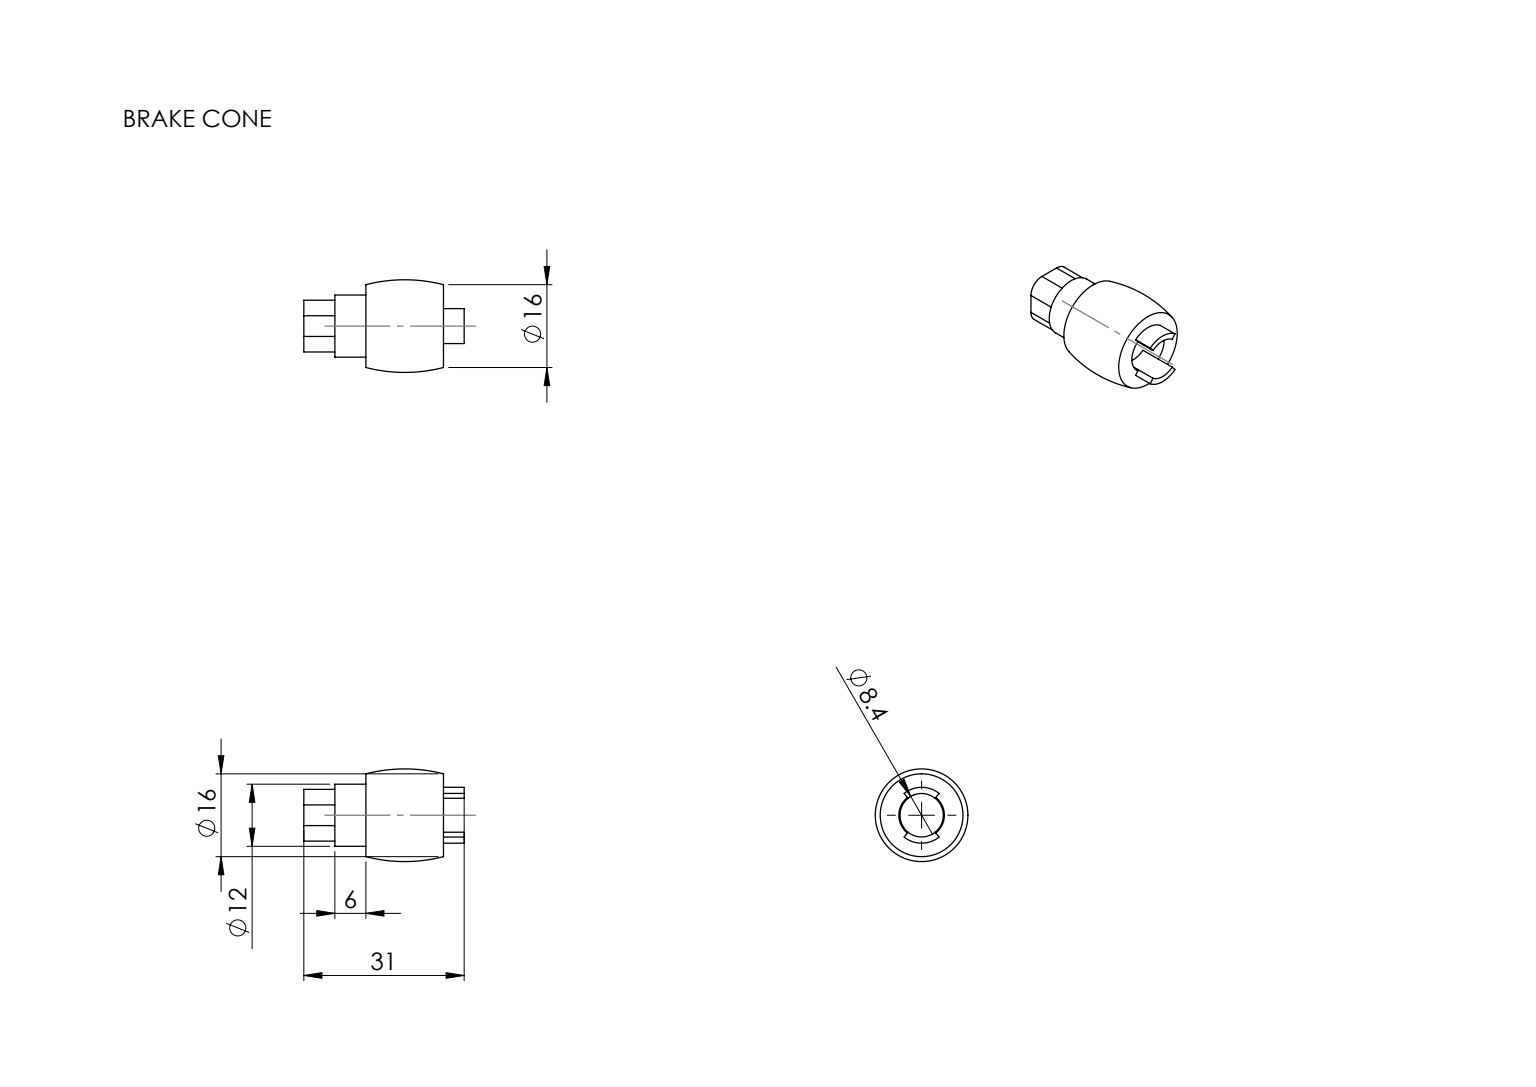
ISO-10303-21;
HEADER;
FILE_DESCRIPTION (('STEP AP214'),
    '1' );
FILE_NAME ('brake cone.step',
    '2026-10-08T05:56:58',
    ( '' ),
    ( '' ),
    'SwSTEP 2.0',
    'SolidWorks 2026',
    '' );
FILE_SCHEMA (( 'AUTOMOTIVE_DESIGN' ));
ENDSEC;

DATA;
#3=AXIS2_PLACEMENT_3D ( 'NONE', #18095, #1186, #4385 ) ;
#13=CARTESIAN_POINT ( 'NONE',  ( -15.00000000000000355, 4.874999999999997335, -3.903123748999000053 ) ) ;
#14=ADVANCED_FACE ( 'NONE', ( #14340, #12840 ), #18938, .T. ) ;
#25=CYLINDRICAL_SURFACE ( 'NONE', #12194, 5.400000000000000355 ) ;
#29=CARTESIAN_POINT ( 'NONE',  ( -41.99999999999999289, -2.000000000000001776, 5.000000000000000000 ) ) ;
#46=VECTOR ( 'NONE', #13444, 1000.000000000000000 ) ;
#90=PLANE ( 'NONE',  #2084 ) ;
#96=ORIENTED_EDGE ( 'NONE', *, *, #17923, .T. ) ;
#107=EDGE_LOOP ( 'NONE', ( #13060, #5147, #11835, #11833, #16317, #5831 ) ) ;
#112=EDGE_LOOP ( 'NONE', ( #14976, #17083 ) ) ;
#123=VERTEX_POINT ( 'NONE', #15646 ) ;
#140=LINE ( 'NONE', #6221, #2071 ) ;
#166=ORIENTED_EDGE ( 'NONE', *, *, #11587, .F. ) ;
#170=EDGE_CURVE ( 'NONE', #2370, #11052, #11954, .T. ) ;
#178=LINE ( 'NONE', #6262, #6325 ) ;
#190=EDGE_CURVE ( 'NONE', #10991, #3279, #7426, .T. ) ;
#207=CARTESIAN_POINT ( 'NONE',  ( -41.99999999999999289, -2.000000000000001776, -2.000000000000000000 ) ) ;
#240=DIRECTION ( 'NONE',  ( 0.000000000000000000, 0.000000000000000000, 1.000000000000000000 ) ) ;
#251=AXIS2_PLACEMENT_3D ( 'NONE', #17536, #9945, #11526 ) ;
#315=ORIENTED_EDGE ( 'NONE', *, *, #13010, .T. ) ;
#337=DIRECTION ( 'NONE',  ( 1.000000000000000000, 6.419766481290786633E-33, -0.000000000000000000 ) ) ;
#348=ORIENTED_EDGE ( 'NONE', *, *, #8508, .T. ) ;
#359=CARTESIAN_POINT ( 'NONE',  ( -11.00000000000000355, -4.215373648918917304, -3.375000000000002665 ) ) ;
#371=ADVANCED_FACE ( 'NONE', ( #7931 ), #17448, .F. ) ;
#385=EDGE_CURVE ( 'NONE', #2370, #813, #18633, .T. ) ;
#410=CIRCLE ( 'NONE', #17678, 5.400000000000000355 ) ;
#413=ADVANCED_FACE ( 'NONE', ( #6417 ), #18643, .T. ) ;
#438=PLANE ( 'NONE',  #10003 ) ;
#452=DIRECTION ( 'NONE',  ( 0.000000000000000000, 1.000000000000000000, 0.000000000000000000 ) ) ;
#464=ORIENTED_EDGE ( 'NONE', *, *, #491, .T. ) ;
#467=AXIS2_PLACEMENT_3D ( 'NONE', #2237, #17453, #19046 ) ;
#470=PLANE ( 'NONE',  #17230 ) ;
#483=DIRECTION ( 'NONE',  ( -1.000000000000000000, -6.419766481290786633E-33, 0.000000000000000000 ) ) ;
#491=EDGE_CURVE ( 'NONE', #14026, #12070, #7010, .T. ) ;
#504=EDGE_CURVE ( 'NONE', #17943, #9399, #4719, .T. ) ;
#516=ORIENTED_EDGE ( 'NONE', *, *, #190, .T. ) ;
#527=EDGE_CURVE ( 'NONE', #16516, #11599, #15232, .T. ) ;
#530=VERTEX_POINT ( 'NONE', #15333 ) ;
#559=FACE_BOUND ( 'NONE', #1659, .T. ) ;
#561=EDGE_LOOP ( 'NONE', ( #1766, #13669, #6712, #18454, #1075, #7563, #16391, #5040 ) ) ;
#565=VECTOR ( 'NONE', #8267, 1000.000000000000000 ) ;
#573=DIRECTION ( 'NONE',  ( 1.000000000000000000, 6.419766481290786633E-33, -0.000000000000000000 ) ) ;
#579=ORIENTED_EDGE ( 'NONE', *, *, #19561, .F. ) ;
#610=ORIENTED_EDGE ( 'NONE', *, *, #19296, .F. ) ;
#617=DIRECTION ( 'NONE',  ( 1.000000000000000000, 6.419766481290786633E-33, -0.000000000000000000 ) ) ;
#640=ADVANCED_FACE ( 'NONE', ( #14022 ), #1910, .T. ) ;
#644=ORIENTED_EDGE ( 'NONE', *, *, #6204, .T. ) ;
#655=ORIENTED_EDGE ( 'NONE', *, *, #19266, .F. ) ;
#702=DIRECTION ( 'NONE',  ( 6.419766481290786633E-33, -1.000000000000000000, 0.000000000000000000 ) ) ;
#708=ORIENTED_EDGE ( 'NONE', *, *, #12930, .T. ) ;
#727=ORIENTED_EDGE ( 'NONE', *, *, #2944, .F. ) ;
#766=SURFACE_STYLE_FILL_AREA ( #5055 ) ;
#767=PRODUCT_DEFINITION_SHAPE ( 'NONE', 'NONE',  #9076 ) ;
#776=EDGE_LOOP ( 'NONE', ( #15679, #8898, #8555, #10719 ) ) ;
#777=EDGE_CURVE ( 'NONE', #2407, #17288, #6813, .T. ) ;
#784=LINE ( 'NONE', #5274, #11574 ) ;
#813=VERTEX_POINT ( 'NONE', #13020 ) ;
#818=DIRECTION ( 'NONE',  ( 1.000000000000000000, 6.419766481290786633E-33, -0.000000000000000000 ) ) ;
#830=FACE_OUTER_BOUND ( 'NONE', #14532, .T. ) ;
#843=ORIENTED_EDGE ( 'NONE', *, *, #491, .F. ) ;
#885=DIRECTION ( 'NONE',  ( 1.000000000000000000, 1.224646799147353207E-16, 0.000000000000000000 ) ) ;
#913=DIRECTION ( 'NONE',  ( -1.000000000000000000, 1.224646799147353207E-16, 0.000000000000000000 ) ) ;
#920=FACE_OUTER_BOUND ( 'NONE', #18601, .T. ) ;
#927=CARTESIAN_POINT ( 'NONE',  ( -11.00000000000000355, 3.278623949159159778, 2.625000000000000888 ) ) ;
#951=ORIENTED_EDGE ( 'NONE', *, *, #13359, .T. ) ;
#952=CARTESIAN_POINT ( 'NONE',  ( -36.00000000000000000, 1.999999999999998224, -5.000000000000000000 ) ) ;
#957=EDGE_LOOP ( 'NONE', ( #10118, #13966, #3448, #4840 ) ) ;
#973=CIRCLE ( 'NONE', #3, 3.000000000000000000 ) ;
#1030=ORIENTED_EDGE ( 'NONE', *, *, #6750, .F. ) ;
#1040=CARTESIAN_POINT ( 'NONE',  ( -10.99900000000000233, 4.200000000000000178, 5.143516556418882928E-16 ) ) ;
#1044=FACE_OUTER_BOUND ( 'NONE', #18531, .T. ) ;
#1075=ORIENTED_EDGE ( 'NONE', *, *, #15150, .T. ) ;
#1083=DIRECTION ( 'NONE',  ( -1.000000000000000000, -1.224646799147353207E-16, 0.000000000000000000 ) ) ;
#1109=CARTESIAN_POINT ( 'NONE',  ( -19.00000000000000355, -4.200000000000000178, 0.000000000000000000 ) ) ;
#1111=ORIENTED_EDGE ( 'NONE', *, *, #11893, .T. ) ;
#1186=DIRECTION ( 'NONE',  ( -1.000000000000000000, 0.000000000000000000, 0.000000000000000000 ) ) ;
#1242=( NAMED_UNIT ( * ) PLANE_ANGLE_UNIT ( ) SI_UNIT ( $, .RADIAN. ) );
#1243=PRODUCT ( 'brake cone', 'brake cone', '', ( #7842 ) ) ;
#1244=VECTOR ( 'NONE', #3600, 1000.000000000000000 ) ;
#1246=LINE ( 'NONE', #7323, #46 ) ;
#1283=ORIENTED_EDGE ( 'NONE', *, *, #10304, .T. ) ;
#1295=EDGE_CURVE ( 'NONE', #5646, #11950, #19297, .T. ) ;
#1330=ORIENTED_EDGE ( 'NONE', *, *, #12486, .F. ) ;
#1362=ORIENTED_EDGE ( 'NONE', *, *, #16739, .T. ) ;
#1371=DIRECTION ( 'NONE',  ( 9.559896011775280412E-17, -0.7806247497997995666, -0.6250000000000001110 ) ) ;
#1395=DIRECTION ( 'NONE',  ( -1.000000000000000000, -6.419766481290788001E-33, -0.000000000000000000 ) ) ;
#1414=EDGE_CURVE ( 'NONE', #16293, #11503, #18340, .T. ) ;
#1469=VECTOR ( 'NONE', #9851, 1000.000000000000114 ) ;
#1491=CARTESIAN_POINT ( 'NONE',  ( -41.99999999999999289, -5.000000000000001776, 5.000000000000000000 ) ) ;
#1493=ORIENTED_EDGE ( 'NONE', *, *, #19398, .T. ) ;
#1508=VECTOR ( 'NONE', #13779, 1000.000000000000000 ) ;
#1516=CARTESIAN_POINT ( 'NONE',  ( -15.00000000000000355, 4.215373648918918192, 3.375000000000000888 ) ) ;
#1534=DIRECTION ( 'NONE',  ( -1.000000000000000000, 1.224646799147353207E-16, 0.000000000000000000 ) ) ;
#1539=CIRCLE ( 'NONE', #12081, 4.200000000000000178 ) ;
#1572=ORIENTED_EDGE ( 'NONE', *, *, #4535, .T. ) ;
#1581=CARTESIAN_POINT ( 'NONE',  ( -36.00000000000000000, 1.999999999999999112, -2.000000000000000000 ) ) ;
#1588=FACE_OUTER_BOUND ( 'NONE', #2951, .T. ) ;
#1623=DIRECTION ( 'NONE',  ( 7.654042494670959086E-17, 0.6250000000000002220, 0.7806247497997996776 ) ) ;
#1659=EDGE_LOOP ( 'NONE', ( #3254, #3461 ) ) ;
#1676=SHAPE_REPRESENTATION_RELATIONSHIP ( 'NONE' , 'NONE' ,  #12077, #3271 ) ;
#1679=LINE ( 'NONE', #3474, #4102 ) ;
#1685=DIRECTION ( 'NONE',  ( -1.000000000000000000, -6.419766481290786633E-33, 0.000000000000000000 ) ) ;
#1693=ADVANCED_FACE ( 'NONE', ( #11331 ), #17129, .F. ) ;
#1716=DIRECTION ( 'NONE',  ( -1.000000000000000000, 1.224646799147353207E-16, 0.000000000000000000 ) ) ;
#1745=ORIENTED_EDGE ( 'NONE', *, *, #18107, .T. ) ;
#1754=LINE ( 'NONE', #13958, #6782 ) ;
#1766=ORIENTED_EDGE ( 'NONE', *, *, #12191, .T. ) ;
#1860=CIRCLE ( 'NONE', #15588, 5.400000000000000355 ) ;
#1867=ORIENTED_EDGE ( 'NONE', *, *, #12851, .F. ) ;
#1870=ORIENTED_EDGE ( 'NONE', *, *, #7757, .T. ) ;
#1882=ORIENTED_EDGE ( 'NONE', *, *, #16897, .T. ) ;
#1887=EDGE_CURVE ( 'NONE', #11052, #6746, #3980, .T. ) ;
#1892=DIRECTION ( 'NONE',  ( -1.000000000000000000, -6.419766481290788001E-33, -0.000000000000000000 ) ) ;
#1902=ORIENTED_EDGE ( 'NONE', *, *, #2961, .T. ) ;
#1907=EDGE_LOOP ( 'NONE', ( #6125, #4723, #348, #7790 ) ) ;
#1910=PLANE ( 'NONE',  #12696 ) ;
#1917=CARTESIAN_POINT ( 'NONE',  ( -11.00000000000000355, 3.278623949159158446, -2.625000000000002220 ) ) ;
#1921=AXIS2_PLACEMENT_3D ( 'NONE', #14124, #1623, #3423 ) ;
#2002=EDGE_CURVE ( 'NONE', #17554, #17936, #16514, .T. ) ;
#2009=VERTEX_POINT ( 'NONE', #8907 ) ;
#2010=AXIS2_PLACEMENT_3D ( 'NONE', #9492, #11283, #11182 ) ;
#2015=LINE ( 'NONE', #14223, #10652 ) ;
#2020=ORIENTED_EDGE ( 'NONE', *, *, #13795, .F. ) ;
#2045=DIRECTION ( 'NONE',  ( -1.000000000000000000, 1.224646799147353207E-16, 0.000000000000000000 ) ) ;
#2061=ORIENTED_EDGE ( 'NONE', *, *, #19767, .F. ) ;
#2065=ORIENTED_EDGE ( 'NONE', *, *, #7779, .F. ) ;
#2071=VECTOR ( 'NONE', #13745, 1000.000000000000000 ) ;
#2076=CARTESIAN_POINT ( 'NONE',  ( -19.00000000000000355, 4.400000000000000355, 0.000000000000000000 ) ) ;
#2084=AXIS2_PLACEMENT_3D ( 'NONE', #7784, #6179, #12691 ) ;
#2122=VECTOR ( 'NONE', #4317, 1000.000000000000000 ) ;
#2130=ADVANCED_FACE ( 'NONE', ( #11197 ), #9711, .F. ) ;
#2152=CIRCLE ( 'NONE', #17170, 5.400000000000000355 ) ;
#2171=CARTESIAN_POINT ( 'NONE',  ( -41.99999999999999289, -1.469576158976823947E-15, 0.000000000000000000 ) ) ;
#2232=ORIENTED_EDGE ( 'NONE', *, *, #11453, .T. ) ;
#2237=CARTESIAN_POINT ( 'NONE',  ( -11.00000000000000355, 4.898587196589412829E-16, 0.000000000000000000 ) ) ;
#2247=ORIENTED_EDGE ( 'NONE', *, *, #19398, .F. ) ;
#2278=AXIS2_PLACEMENT_3D ( 'NONE', #13838, #18436, #19734 ) ;
#2282=DIRECTION ( 'NONE',  ( 1.000000000000000000, 6.419766481290786633E-33, -0.000000000000000000 ) ) ;
#2291=AXIS2_PLACEMENT_3D ( 'NONE', #6294, #6200, #11114 ) ;
#2347=DIRECTION ( 'NONE',  ( 0.000000000000000000, -1.000000000000000000, 0.000000000000000000 ) ) ;
#2365=VERTEX_POINT ( 'NONE', #9087 ) ;
#2370=VERTEX_POINT ( 'NONE', #12181 ) ;
#2407=VERTEX_POINT ( 'NONE', #8786 ) ;
#2413=AXIS2_PLACEMENT_3D ( 'NONE', #11245, #7837, #4842 ) ;
#2460=DIRECTION ( 'NONE',  ( -1.000000000000000000, 0.000000000000000000, 0.000000000000000000 ) ) ;
#2468=DIRECTION ( 'NONE',  ( 0.000000000000000000, 1.000000000000000000, 0.000000000000000000 ) ) ;
#2479=CIRCLE ( 'NONE', #251, 30.00000000000000355 ) ;
#2491=AXIS2_PLACEMENT_3D ( 'NONE', #6337, #3251, #18656 ) ;
#2508=AXIS2_PLACEMENT_3D ( 'NONE', #4240, #10254, #2629 ) ;
#2511=PLANE ( 'NONE',  #16664 ) ;
#2516=FACE_OUTER_BOUND ( 'NONE', #16831, .T. ) ;
#2525=DIRECTION ( 'NONE',  ( 1.000000000000000000, 6.419766481290786633E-33, -0.000000000000000000 ) ) ;
#2539=ORIENTED_EDGE ( 'NONE', *, *, #7560, .T. ) ;
#2548=ORIENTED_EDGE ( 'NONE', *, *, #15430, .F. ) ;
#2628=DIRECTION ( 'NONE',  ( -1.000000000000000000, -6.419766481290788001E-33, -0.000000000000000000 ) ) ;
#2629=DIRECTION ( 'NONE',  ( 0.000000000000000000, -1.000000000000000000, 0.000000000000000000 ) ) ;
#2739=CARTESIAN_POINT ( 'NONE',  ( -30.00000000000000000, 8.000000000000000000, 0.000000000000000000 ) ) ;
#2792=DIRECTION ( 'NONE',  ( -9.559896011775280412E-17, -0.7806247497997995666, -0.6250000000000002220 ) ) ;
#2839=DIRECTION ( 'NONE',  ( -1.000000000000000000, -1.224646799147353207E-16, -0.000000000000000000 ) ) ;
#2871=ORIENTED_EDGE ( 'NONE', *, *, #19538, .F. ) ;
#2889=EDGE_CURVE ( 'NONE', #123, #9264, #1754, .T. ) ;
#2891=PLANE ( 'NONE',  #3067 ) ;
#2905=AXIS2_PLACEMENT_3D ( 'NONE', #15793, #8184, #13348 ) ;
#2933=ADVANCED_FACE ( 'NONE', ( #559, #3747 ), #6928, .T. ) ;
#2944=EDGE_CURVE ( 'NONE', #12101, #5745, #3928, .T. ) ;
#2951=EDGE_LOOP ( 'NONE', ( #1493, #13570, #18839, #2548, #13326, #16612 ) ) ;
#2961=EDGE_CURVE ( 'NONE', #17554, #3802, #14354, .T. ) ;
#2972=DIRECTION ( 'NONE',  ( -1.000000000000000000, -6.419766481290786633E-33, 0.000000000000000000 ) ) ;
#3019=VERTEX_POINT ( 'NONE', #6092 ) ;
#3067=AXIS2_PLACEMENT_3D ( 'NONE', #10511, #19606, #13503 ) ;
#3085=CIRCLE ( 'NONE', #14277, 3.000000000000000000 ) ;
#3105=CARTESIAN_POINT ( 'NONE',  ( -41.99999999999999289, 1.999999999999998224, -2.000000000000000000 ) ) ;
#3137=CARTESIAN_POINT ( 'NONE',  ( -19.00000000000000355, 3.278623949159158890, 2.625000000000000888 ) ) ;
#3142=CIRCLE ( 'NONE', #16246, 3.000000000000000000 ) ;
#3170=( NAMED_UNIT ( * ) PLANE_ANGLE_UNIT ( ) SI_UNIT ( $, .RADIAN. ) );
#3173=EDGE_LOOP ( 'NONE', ( #1745, #9621 ) ) ;
#3204=TOROIDAL_SURFACE ( 'NONE', #13424, -21.04737509655562988, 30.00000000000000355 ) ;
#3222=VERTEX_POINT ( 'NONE', #10297 ) ;
#3251=DIRECTION ( 'NONE',  ( -1.000000000000000000, 1.224646799147353207E-16, 0.000000000000000000 ) ) ;
#3254=ORIENTED_EDGE ( 'NONE', *, *, #10304, .F. ) ;
#3257=EDGE_LOOP ( 'NONE', ( #4050, #7202 ) ) ;
#3271=ADVANCED_BREP_SHAPE_REPRESENTATION ( '', ( #9200, #16724 ), #3651 ) ;
#3279=VERTEX_POINT ( 'NONE', #10008 ) ;
#3294=AXIS2_PLACEMENT_3D ( 'NONE', #3737, #8138, #15948 ) ;
#3301=CARTESIAN_POINT ( 'NONE',  ( -36.00000000000000000, -2.000000000000000888, -2.000000000000000000 ) ) ;
#3312=ORIENTED_EDGE ( 'NONE', *, *, #8331, .T. ) ;
#3322=DIRECTION ( 'NONE',  ( 1.000000000000000000, 6.419766481290786633E-33, -0.000000000000000000 ) ) ;
#3327=ORIENTED_EDGE ( 'NONE', *, *, #5451, .F. ) ;
#3379=CIRCLE ( 'NONE', #14252, 4.400000000000000355 ) ;
#3416=CARTESIAN_POINT ( 'NONE',  ( -19.00000000000000355, -4.898587196589412829E-16, 0.000000000000000000 ) ) ;
#3423=DIRECTION ( 'NONE',  ( 0.000000000000000000, -0.7806247497997995666, 0.6250000000000001110 ) ) ;
#3438=VECTOR ( 'NONE', #5443, 1000.000000000000000 ) ;
#3439=DIRECTION ( 'NONE',  ( 6.419766481290786633E-33, -1.000000000000000000, 0.000000000000000000 ) ) ;
#3440=DIRECTION ( 'NONE',  ( 0.000000000000000000, 1.000000000000000000, 0.000000000000000000 ) ) ;
#3442=ORIENTED_EDGE ( 'NONE', *, *, #8852, .T. ) ;
#3448=ORIENTED_EDGE ( 'NONE', *, *, #18107, .F. ) ;
#3458=EDGE_CURVE ( 'NONE', #3222, #14330, #2152, .T. ) ;
#3461=ORIENTED_EDGE ( 'NONE', *, *, #13010, .F. ) ;
#3469=SURFACE_STYLE_USAGE ( .BOTH. , #14173 ) ;
#3474=CARTESIAN_POINT ( 'NONE',  ( -41.99999999999999289, -5.000000000000001776, -2.000000000000000000 ) ) ;
#3478=PRODUCT_DEFINITION_FORMATION_WITH_SPECIFIED_SOURCE ( 'ANY', '', #1243, .NOT_KNOWN. ) ;
#3492=EDGE_LOOP ( 'NONE', ( #1111, #2539, #14378, #7011, #7147, #2065 ) ) ;
#3509=EDGE_LOOP ( 'NONE', ( #2020, #10777, #464, #19765 ) ) ;
#3535=CARTESIAN_POINT ( 'NONE',  ( -41.99999999999999289, -2.000000000000001776, 2.000000000000000000 ) ) ;
#3540=ORIENTED_EDGE ( 'NONE', *, *, #5764, .F. ) ;
#3566=CARTESIAN_POINT ( 'NONE',  ( -30.00000000000000000, -1.925929944387235853E-31, 0.000000000000000000 ) ) ;
#3572=ORIENTED_EDGE ( 'NONE', *, *, #17156, .T. ) ;
#3600=DIRECTION ( 'NONE',  ( -1.000000000000000000, -1.224646799147353207E-16, 0.000000000000000000 ) ) ;
#3616=VERTEX_POINT ( 'NONE', #12934 ) ;
#3619=DIRECTION ( 'NONE',  ( 0.000000000000000000, 1.000000000000000000, 0.000000000000000000 ) ) ;
#3637=CARTESIAN_POINT ( 'NONE',  ( -15.00000000000000355, -4.215373648918917304, -3.375000000000002220 ) ) ;
#3638=ADVANCED_FACE ( 'NONE', ( #830 ), #11718, .F. ) ;
#3651=( GEOMETRIC_REPRESENTATION_CONTEXT ( 3 ) GLOBAL_UNCERTAINTY_ASSIGNED_CONTEXT ( ( #19587 ) ) GLOBAL_UNIT_ASSIGNED_CONTEXT ( ( #4281, #8785, #13380 ) ) REPRESENTATION_CONTEXT ( 'NONE', 'WORKASPACE' ) );
#3673=FACE_OUTER_BOUND ( 'NONE', #17019, .T. ) ;
#3728=VERTEX_POINT ( 'NONE', #8914 ) ;
#3737=CARTESIAN_POINT ( 'NONE',  ( -10.99900000000000233, -7.061101152771736665E-32, 0.000000000000000000 ) ) ;
#3747=FACE_OUTER_BOUND ( 'NONE', #18882, .T. ) ;
#3753=AXIS2_PLACEMENT_3D ( 'NONE', #10349, #5919, #19434 ) ;
#3758=CARTESIAN_POINT ( 'NONE',  ( -36.00000000000000000, -6.000000000000000888, 7.347880794884120722E-16 ) ) ;
#3759=ORIENTED_EDGE ( 'NONE', *, *, #4413, .F. ) ;
#3769=ORIENTED_EDGE ( 'NONE', *, *, #16974, .T. ) ;
#3780=CYLINDRICAL_SURFACE ( 'NONE', #2905, 4.200000000000000178 ) ;
#3802=VERTEX_POINT ( 'NONE', #18699 ) ;
#3815=ORIENTED_EDGE ( 'NONE', *, *, #777, .T. ) ;
#3891=CARTESIAN_POINT ( 'NONE',  ( -36.00000000000000000, -5.000000000000000888, 5.000000000000000000 ) ) ;
#3900=EDGE_CURVE ( 'NONE', #11206, #6326, #15709, .T. ) ;
#3916=CARTESIAN_POINT ( 'NONE',  ( -15.00000000000000355, 1.224646799147353454E-16, 0.000000000000000000 ) ) ;
#3928=CIRCLE ( 'NONE', #5190, 4.200000000000000178 ) ;
#3940=AXIS2_PLACEMENT_3D ( 'NONE', #3535, #17151, #4944 ) ;
#3980=CIRCLE ( 'NONE', #17723, 4.200000000000000178 ) ;
#3981=CARTESIAN_POINT ( 'NONE',  ( -41.99999999999999289, -3.184081677783117402E-15, 0.000000000000000000 ) ) ;
#4004=AXIS2_PLACEMENT_3D ( 'NONE', #16285, #11677, #8778 ) ;
#4025=EDGE_LOOP ( 'NONE', ( #11265, #15956, #13762, #7318 ) ) ;
#4047=DIRECTION ( 'NONE',  ( 0.000000000000000000, -1.000000000000000000, 0.000000000000000000 ) ) ;
#4050=ORIENTED_EDGE ( 'NONE', *, *, #12191, .F. ) ;
#4071=VERTEX_POINT ( 'NONE', #10965 ) ;
#4078=AXIS2_PLACEMENT_3D ( 'NONE', #17849, #4144, #10256 ) ;
#4093=VECTOR ( 'NONE', #9042, 1000.000000000000000 ) ;
#4102=VECTOR ( 'NONE', #14075, 1000.000000000000000 ) ;
#4142=CARTESIAN_POINT ( 'NONE',  ( -36.00000000000000000, -2.311115933264683024E-31, 0.000000000000000000 ) ) ;
#4144=DIRECTION ( 'NONE',  ( 1.000000000000000000, 6.419766481290786633E-33, -0.000000000000000000 ) ) ;
#4145=ORIENTED_EDGE ( 'NONE', *, *, #11453, .F. ) ;
#4199=EDGE_CURVE ( 'NONE', #813, #6746, #6935, .T. ) ;
#4240=CARTESIAN_POINT ( 'NONE',  ( -19.00000000000000355, 1.224646799147353207E-16, 0.000000000000000000 ) ) ;
#4248=AXIS2_PLACEMENT_3D ( 'NONE', #6038, #12159, #7134 ) ;
#4277=ADVANCED_FACE ( 'NONE', ( #17658 ), #11842, .F. ) ;
#4278=EDGE_CURVE ( 'NONE', #11503, #4614, #16254, .T. ) ;
#4281=( LENGTH_UNIT ( ) NAMED_UNIT ( * ) SI_UNIT ( .MILLI., .METRE. ) );
#4296=VECTOR ( 'NONE', #2792, 1000.000000000000000 ) ;
#4307=CARTESIAN_POINT ( 'NONE',  ( -36.00000000000000000, 6.000000000000000888, 0.000000000000000000 ) ) ;
#4317=DIRECTION ( 'NONE',  ( -1.000000000000000000, -1.224646799147353207E-16, 0.000000000000000000 ) ) ;
#4323=ADVANCED_FACE ( 'NONE', ( #1044 ), #11748, .T. ) ;
#4330=ORIENTED_EDGE ( 'NONE', *, *, #4278, .F. ) ;
#4334=VECTOR ( 'NONE', #14147, 1000.000000000000000 ) ;
#4354=FACE_OUTER_BOUND ( 'NONE', #3257, .T. ) ;
#4375=DIRECTION ( 'NONE',  ( 0.000000000000000000, -1.000000000000000000, 0.000000000000000000 ) ) ;
#4385=DIRECTION ( 'NONE',  ( 0.000000000000000000, 0.000000000000000000, 1.000000000000000000 ) ) ;
#4400=CARTESIAN_POINT ( 'NONE',  ( -36.00000000000000000, -2.000000000000000888, -5.000000000000000000 ) ) ;
#4413=EDGE_CURVE ( 'NONE', #10153, #12571, #7827, .T. ) ;
#4430=VERTEX_POINT ( 'NONE', #12147 ) ;
#4451=PLANE ( 'NONE',  #9050 ) ;
#4463=ORIENTED_EDGE ( 'NONE', *, *, #1887, .T. ) ;
#4497=AXIS2_PLACEMENT_3D ( 'NONE', #10023, #19014, #18910 ) ;
#4499=DIRECTION ( 'NONE',  ( 0.000000000000000000, -3.552713678800500929E-15, 1.000000000000000000 ) ) ;
#4508=VECTOR ( 'NONE', #9052, 1000.000000000000000 ) ;
#4525=DIRECTION ( 'NONE',  ( 0.000000000000000000, -1.000000000000000000, 0.000000000000000000 ) ) ;
#4535=EDGE_CURVE ( 'NONE', #12710, #9399, #1539, .T. ) ;
#4556=ORIENTED_EDGE ( 'NONE', *, *, #13741, .F. ) ;
#4561=EDGE_CURVE ( 'NONE', #2407, #6506, #2479, .T. ) ;
#4605=VERTEX_POINT ( 'NONE', #19511 ) ;
#4614=VERTEX_POINT ( 'NONE', #1516 ) ;
#4631=DIRECTION ( 'NONE',  ( 0.000000000000000000, 0.000000000000000000, 1.000000000000000000 ) ) ;
#4633=DIRECTION ( 'NONE',  ( -1.000000000000000000, -6.419766481290786633E-33, 0.000000000000000000 ) ) ;
#4641=CYLINDRICAL_SURFACE ( 'NONE', #13787, 5.400000000000000355 ) ;
#4679=DIRECTION ( 'NONE',  ( 1.000000000000000000, 6.419766481290786633E-33, -0.000000000000000000 ) ) ;
#4688=AXIS2_PLACEMENT_3D ( 'NONE', #14400, #17296, #9808 ) ;
#4711=EDGE_LOOP ( 'NONE', ( #6255, #5433 ) ) ;
#4719=LINE ( 'NONE', #15029, #14493 ) ;
#4723=ORIENTED_EDGE ( 'NONE', *, *, #18434, .T. ) ;
#4756=CIRCLE ( 'NONE', #17547, 4.400000000000000355 ) ;
#4776=DIRECTION ( 'NONE',  ( -1.000000000000000000, -1.224646799147353207E-16, 0.000000000000000000 ) ) ;
#4777=DIRECTION ( 'NONE',  ( 0.000000000000000000, 1.000000000000000000, 0.000000000000000000 ) ) ;
#4799=DIRECTION ( 'NONE',  ( -1.000000000000000000, 1.224646799147353207E-16, 0.000000000000000000 ) ) ;
#4808=DIRECTION ( 'NONE',  ( 1.000000000000000000, 6.419766481290786633E-33, -0.000000000000000000 ) ) ;
#4824=EDGE_CURVE ( 'NONE', #16982, #4071, #17213, .T. ) ;
#4840=ORIENTED_EDGE ( 'NONE', *, *, #9198, .F. ) ;
#4842=DIRECTION ( 'NONE',  ( 0.000000000000000000, 0.000000000000000000, 1.000000000000000000 ) ) ;
#4860=VECTOR ( 'NONE', #15503, 1000.000000000000000 ) ;
#4907=DIRECTION ( 'NONE',  ( 0.000000000000000000, 1.000000000000000000, 0.000000000000000000 ) ) ;
#4917=VERTEX_POINT ( 'NONE', #14701 ) ;
#4919=AXIS2_PLACEMENT_3D ( 'NONE', #11244, #17350, #17549 ) ;
#4927=FACE_OUTER_BOUND ( 'NONE', #19728, .T. ) ;
#4944=DIRECTION ( 'NONE',  ( 0.000000000000000000, 1.000000000000000000, 0.000000000000000000 ) ) ;
#4949=CARTESIAN_POINT ( 'NONE',  ( -41.99999999999999289, 1.999999999999998224, 2.000000000000000000 ) ) ;
#4963=VERTEX_POINT ( 'NONE', #18199 ) ;
#5034=EDGE_CURVE ( 'NONE', #9172, #2365, #12094, .T. ) ;
#5039=CARTESIAN_POINT ( 'NONE',  ( -41.99999999999999289, 4.999999999999998224, 2.000000000000000000 ) ) ;
#5040=ORIENTED_EDGE ( 'NONE', *, *, #3900, .F. ) ;
#5055=FILL_AREA_STYLE ('',( #12767 ) ) ;
#5073=DIRECTION ( 'NONE',  ( -1.000000000000000000, -1.224646799147353207E-16, -0.000000000000000000 ) ) ;
#5101=DIRECTION ( 'NONE',  ( 1.000000000000000000, 6.419766481290786633E-33, -0.000000000000000000 ) ) ;
#5121=CARTESIAN_POINT ( 'NONE',  ( -11.00000000000000355, -4.215373648918918192, 3.375000000000000888 ) ) ;
#5130=FACE_OUTER_BOUND ( 'NONE', #776, .T. ) ;
#5131=FACE_OUTER_BOUND ( 'NONE', #7335, .T. ) ;
#5146=SURFACE_SIDE_STYLE ('',( #766 ) ) ;
#5147=ORIENTED_EDGE ( 'NONE', *, *, #13235, .T. ) ;
#5176=ADVANCED_FACE ( 'NONE', ( #6657, #3673 ), #11285, .T. ) ;
#5189=LINE ( 'NONE', #11307, #10570 ) ;
#5190=AXIS2_PLACEMENT_3D ( 'NONE', #5437, #14257, #12956 ) ;
#5216=CARTESIAN_POINT ( 'NONE',  ( -30.00000000000000000, 1.224646799147352468E-16, 0.000000000000000000 ) ) ;
#5230=CARTESIAN_POINT ( 'NONE',  ( -36.00000000000000000, -2.311115933264683024E-31, 0.000000000000000000 ) ) ;
#5258=CARTESIAN_POINT ( 'NONE',  ( -15.00000000000000355, 8.000000000000000000, 0.000000000000000000 ) ) ;
#5268=DIRECTION ( 'NONE',  ( 0.000000000000000000, -1.000000000000000000, 0.000000000000000000 ) ) ;
#5274=CARTESIAN_POINT ( 'NONE',  ( -41.99999999999999289, -5.000000000000001776, 2.000000000000000000 ) ) ;
#5299=EDGE_CURVE ( 'NONE', #4071, #10940, #3379, .T. ) ;
#5356=DIRECTION ( 'NONE',  ( 1.000000000000000000, 6.419766481290786633E-33, -0.000000000000000000 ) ) ;
#5388=UNCERTAINTY_MEASURE_WITH_UNIT (LENGTH_MEASURE( 1.000000000000000082E-05 ), #9778, 'distance_accuracy_value', 'NONE');
#5391=LINE ( 'NONE', #3891, #8926 ) ;
#5393=DIRECTION ( 'NONE',  ( 0.000000000000000000, 1.000000000000000000, 0.000000000000000000 ) ) ;
#5411=CARTESIAN_POINT ( 'NONE',  ( -36.00000000000000000, 4.200000000000000178, 5.143516556418882928E-16 ) ) ;
#5421=EDGE_LOOP ( 'NONE', ( #13302, #6886, #10808, #3540 ) ) ;
#5433=ORIENTED_EDGE ( 'NONE', *, *, #18434, .F. ) ;
#5437=CARTESIAN_POINT ( 'NONE',  ( -36.00000000000000000, -2.311115933264683024E-31, 0.000000000000000000 ) ) ;
#5443=DIRECTION ( 'NONE',  ( -1.000000000000000000, -1.224646799147353207E-16, 0.000000000000000000 ) ) ;
#5451=EDGE_CURVE ( 'NONE', #11752, #813, #18733, .T. ) ;
#5485=VERTEX_POINT ( 'NONE', #6611 ) ;
#5496=EDGE_CURVE ( 'NONE', #11752, #530, #16145, .T. ) ;
#5501=FACE_BOUND ( 'NONE', #12681, .T. ) ;
#5511=VECTOR ( 'NONE', #15379, 1000.000000000000000 ) ;
#5522=CARTESIAN_POINT ( 'NONE',  ( -41.99999999999999289, -5.000000000000001776, 5.000000000000000000 ) ) ;
#5535=FACE_OUTER_BOUND ( 'NONE', #107, .T. ) ;
#5540=CARTESIAN_POINT ( 'NONE',  ( -11.00000000000000355, -4.898587196589412829E-16, 0.000000000000000000 ) ) ;
#5601=DIRECTION ( 'NONE',  ( -1.000000000000000000, 0.000000000000000000, -0.000000000000000000 ) ) ;
#5612=CARTESIAN_POINT ( 'NONE',  ( -11.00000000000000355, -4.898587196589412829E-16, 0.000000000000000000 ) ) ;
#5646=VERTEX_POINT ( 'NONE', #7197 ) ;
#5664=FACE_OUTER_BOUND ( 'NONE', #561, .T. ) ;
#5676=CARTESIAN_POINT ( 'NONE',  ( -36.00000000000000000, -5.000000000000000888, 2.000000000000000000 ) ) ;
#5739=DIRECTION ( 'NONE',  ( 6.419766481290786633E-33, -1.000000000000000000, 0.000000000000000000 ) ) ;
#5745=VERTEX_POINT ( 'NONE', #10622 ) ;
#5747=DIRECTION ( 'NONE',  ( 0.000000000000000000, 0.000000000000000000, 1.000000000000000000 ) ) ;
#5764=EDGE_CURVE ( 'NONE', #11950, #8225, #13720, .T. ) ;
#5778=DIRECTION ( 'NONE',  ( -1.000000000000000000, 0.000000000000000000, 0.000000000000000000 ) ) ;
#5779=ORIENTED_EDGE ( 'NONE', *, *, #18937, .F. ) ;
#5805=AXIS2_PLACEMENT_3D ( 'NONE', #11418, #818, #9929 ) ;
#5828=AXIS2_PLACEMENT_3D ( 'NONE', #5230, #11347, #3439 ) ;
#5831=ORIENTED_EDGE ( 'NONE', *, *, #10428, .F. ) ;
#5843=FACE_BOUND ( 'NONE', #4711, .T. ) ;
#5866=LINE ( 'NONE', #9180, #11037 ) ;
#5907=CARTESIAN_POINT ( 'NONE',  ( -41.99999999999999289, 1.999999999999998224, 5.000000000000000000 ) ) ;
#5919=DIRECTION ( 'NONE',  ( 1.000000000000000000, 6.419766481290786633E-33, -0.000000000000000000 ) ) ;
#5969=CARTESIAN_POINT ( 'NONE',  ( -41.99999999999999289, -4.400000000000004796, 5.388445916248358943E-16 ) ) ;
#5993=LINE ( 'NONE', #4307, #8876 ) ;
#6019=ORIENTED_EDGE ( 'NONE', *, *, #18502, .F. ) ;
#6031=EDGE_LOOP ( 'NONE', ( #5779, #2061, #6516, #4145, #8122, #6642 ) ) ;
#6033=CARTESIAN_POINT ( 'NONE',  ( -11.00000000000000355, -4.898587196589412829E-16, 0.000000000000000000 ) ) ;
#6038=CARTESIAN_POINT ( 'NONE',  ( -41.99999999999999289, -3.184081677783117402E-15, 0.000000000000000000 ) ) ;
#6053=ORIENTED_EDGE ( 'NONE', *, *, #6407, .T. ) ;
#6059=DIRECTION ( 'NONE',  ( 0.000000000000000000, -1.000000000000000000, 0.000000000000000000 ) ) ;
#6066=VECTOR ( 'NONE', #15533, 1000.000000000000000 ) ;
#6076=LINE ( 'NONE', #1491, #19375 ) ;
#6092=CARTESIAN_POINT ( 'NONE',  ( -11.00000000000000355, 3.278623949159158446, -2.625000000000002220 ) ) ;
#6094=EDGE_CURVE ( 'NONE', #8225, #10153, #6076, .T. ) ;
#6125=ORIENTED_EDGE ( 'NONE', *, *, #6631, .F. ) ;
#6138=VECTOR ( 'NONE', #14609, 1000.000000000000000 ) ;
#6139=ORIENTED_EDGE ( 'NONE', *, *, #7571, .T. ) ;
#6162=CIRCLE ( 'NONE', #4248, 4.400000000000001243 ) ;
#6165=LINE ( 'NONE', #19773, #6595 ) ;
#6169=DIRECTION ( 'NONE',  ( -1.000000000000000000, 1.224646799147353207E-16, 0.000000000000000000 ) ) ;
#6175=ORIENTED_EDGE ( 'NONE', *, *, #385, .F. ) ;
#6179=DIRECTION ( 'NONE',  ( 7.654042494670960318E-17, 0.6250000000000002220, -0.7806247497997995666 ) ) ;
#6200=DIRECTION ( 'NONE',  ( 1.000000000000000000, 6.419766481290786633E-33, -0.000000000000000000 ) ) ;
#6202=AXIS2_PLACEMENT_3D ( 'NONE', #4949, #8034, #452 ) ;
#6204=EDGE_CURVE ( 'NONE', #17967, #123, #3085, .T. ) ;
#6217=( GEOMETRIC_REPRESENTATION_CONTEXT ( 3 ) GLOBAL_UNCERTAINTY_ASSIGNED_CONTEXT ( ( #5388 ) ) GLOBAL_UNIT_ASSIGNED_CONTEXT ( ( #9778, #1242, #10261 ) ) REPRESENTATION_CONTEXT ( 'NONE', 'WORKASPACE' ) );
#6219=EDGE_LOOP ( 'NONE', ( #1030, #727 ) ) ;
#6221=CARTESIAN_POINT ( 'NONE',  ( -41.99999999999999289, 4.999999999999998224, 5.000000000000000000 ) ) ;
#6225=DIRECTION ( 'NONE',  ( -1.000000000000000000, 1.224646799147353207E-16, 0.000000000000000000 ) ) ;
#6229=DIRECTION ( 'NONE',  ( -1.000000000000000000, 1.224646799147353207E-16, 0.000000000000000000 ) ) ;
#6230=DIRECTION ( 'NONE',  ( 1.000000000000000000, 0.000000000000000000, 0.000000000000000000 ) ) ;
#6255=ORIENTED_EDGE ( 'NONE', *, *, #11780, .F. ) ;
#6259=VECTOR ( 'NONE', #1371, 1000.000000000000114 ) ;
#6262=CARTESIAN_POINT ( 'NONE',  ( -11.00000000000000355, 3.278623949159158446, -2.625000000000002220 ) ) ;
#6265=CARTESIAN_POINT ( 'NONE',  ( -15.00000000000000355, -4.400000000000000355, 5.388445916248354013E-16 ) ) ;
#6288=VECTOR ( 'NONE', #9969, 1000.000000000000000 ) ;
#6294=CARTESIAN_POINT ( 'NONE',  ( -30.00000000000000000, 1.224646799147352468E-16, 0.000000000000000000 ) ) ;
#6325=VECTOR ( 'NONE', #4776, 1000.000000000000000 ) ;
#6326=VERTEX_POINT ( 'NONE', #2076 ) ;
#6329=EDGE_LOOP ( 'NONE', ( #19166, #3815, #15696, #6019 ) ) ;
#6335=ORIENTED_EDGE ( 'NONE', *, *, #8508, .F. ) ;
#6337=CARTESIAN_POINT ( 'NONE',  ( -19.00000000000000355, 1.224646799147353207E-16, 0.000000000000000000 ) ) ;
#6347=LINE ( 'NONE', #7857, #9353 ) ;
#6381=EDGE_LOOP ( 'NONE', ( #16444, #13913, #17642, #16904 ) ) ;
#6407=EDGE_CURVE ( 'NONE', #11503, #8180, #11578, .T. ) ;
#6417=FACE_OUTER_BOUND ( 'NONE', #18974, .T. ) ;
#6450=AXIS2_PLACEMENT_3D ( 'NONE', #10389, #19768, #4375 ) ;
#6458=VECTOR ( 'NONE', #2045, 1000.000000000000000 ) ;
#6506=VERTEX_POINT ( 'NONE', #19338 ) ;
#6510=CARTESIAN_POINT ( 'NONE',  ( -30.00000000000000000, -1.925929944387235853E-31, 0.000000000000000000 ) ) ;
#6516=ORIENTED_EDGE ( 'NONE', *, *, #504, .T. ) ;
#6542=CARTESIAN_POINT ( 'NONE',  ( -41.99999999999999289, -5.000000000000001776, 5.000000000000000000 ) ) ;
#6549=ORIENTED_EDGE ( 'NONE', *, *, #3458, .F. ) ;
#6595=VECTOR ( 'NONE', #2972, 1000.000000000000000 ) ;
#6601=LINE ( 'NONE', #15631, #6066 ) ;
#6603=PLANE ( 'NONE',  #9193 ) ;
#6611=CARTESIAN_POINT ( 'NONE',  ( -36.00000000000000000, 4.400000000000000355, 0.000000000000000000 ) ) ;
#6631=EDGE_CURVE ( 'NONE', #3616, #12101, #13054, .T. ) ;
#6642=ORIENTED_EDGE ( 'NONE', *, *, #4278, .T. ) ;
#6644=DIRECTION ( 'NONE',  ( 0.000000000000000000, 1.000000000000000000, 0.000000000000000000 ) ) ;
#6657=FACE_BOUND ( 'NONE', #112, .T. ) ;
#6658=ADVANCED_FACE ( 'NONE', ( #5535 ), #11643, .T. ) ;
#6659=VERTEX_POINT ( 'NONE', #7721 ) ;
#6697=DIRECTION ( 'NONE',  ( 1.000000000000000000, 6.419766481290786633E-33, -0.000000000000000000 ) ) ;
#6700=ADVANCED_FACE ( 'NONE', ( #18145 ), #25, .T. ) ;
#6712=ORIENTED_EDGE ( 'NONE', *, *, #13235, .F. ) ;
#6746=VERTEX_POINT ( 'NONE', #16642 ) ;
#6750=EDGE_CURVE ( 'NONE', #5745, #12101, #18900, .T. ) ;
#6782=VECTOR ( 'NONE', #12457, 1000.000000000000000 ) ;
#6783=DIRECTION ( 'NONE',  ( 0.000000000000000000, 0.000000000000000000, -1.000000000000000000 ) ) ;
#6813=CIRCLE ( 'NONE', #12900, 8.000000000000000000 ) ;
#6831=CARTESIAN_POINT ( 'NONE',  ( -30.00000000000000000, 4.400000000000000355, 0.000000000000000000 ) ) ;
#6840=SURFACE_STYLE_USAGE ( .BOTH. , #5146 ) ;
#6843=EDGE_LOOP ( 'NONE', ( #19008, #15654, #951, #10598, #1572 ) ) ;
#6854=LINE ( 'NONE', #12982, #10953 ) ;
#6863=DIRECTION ( 'NONE',  ( 0.000000000000000000, 0.7806247497997995666, 0.6250000000000001110 ) ) ;
#6886=ORIENTED_EDGE ( 'NONE', *, *, #10431, .F. ) ;
#6892=CARTESIAN_POINT ( 'NONE',  ( -30.00000000000000000, 1.224646799147352468E-16, 0.000000000000000000 ) ) ;
#6928=PLANE ( 'NONE',  #16382 ) ;
#6935=LINE ( 'NONE', #19246, #6288 ) ;
#6984=ORIENTED_EDGE ( 'NONE', *, *, #7571, .F. ) ;
#7010=LINE ( 'NONE', #5522, #10970 ) ;
#7011=ORIENTED_EDGE ( 'NONE', *, *, #5451, .T. ) ;
#7018=DIRECTION ( 'NONE',  ( 0.000000000000000000, 1.000000000000000000, 0.000000000000000000 ) ) ;
#7041=ORIENTED_EDGE ( 'NONE', *, *, #1295, .T. ) ;
#7077=AXIS2_PLACEMENT_3D ( 'NONE', #11974, #19270, #14977 ) ;
#7102=VECTOR ( 'NONE', #2839, 1000.000000000000000 ) ;
#7134=DIRECTION ( 'NONE',  ( 0.000000000000000000, 1.000000000000000000, 0.000000000000000000 ) ) ;
#7147=ORIENTED_EDGE ( 'NONE', *, *, #4199, .T. ) ;
#7153=ADVANCED_FACE ( 'NONE', ( #14106 ), #18224, .T. ) ;
#7197=CARTESIAN_POINT ( 'NONE',  ( -36.00000000000000000, 4.999999999999999112, 2.000000000000000000 ) ) ;
#7200=DIRECTION ( 'NONE',  ( 0.000000000000000000, -1.000000000000000000, 0.000000000000000000 ) ) ;
#7202=ORIENTED_EDGE ( 'NONE', *, *, #11176, .F. ) ;
#7210=ORIENTED_EDGE ( 'NONE', *, *, #4535, .F. ) ;
#7259=AXIS2_PLACEMENT_3D ( 'NONE', #3301, #9607, #15512 ) ;
#7260=ADVANCED_FACE ( 'NONE', ( #14012 ), #17017, .T. ) ;
#7291=CIRCLE ( 'NONE', #2508, 4.400000000000000355 ) ;
#7307=ORIENTED_EDGE ( 'NONE', *, *, #2889, .F. ) ;
#7313=CARTESIAN_POINT ( 'NONE',  ( -11.00000000000000355, 4.898587196589412829E-16, 0.000000000000000000 ) ) ;
#7318=ORIENTED_EDGE ( 'NONE', *, *, #4413, .T. ) ;
#7323=CARTESIAN_POINT ( 'NONE',  ( -36.00000000000000000, -5.000000000000001776, -5.000000000000000000 ) ) ;
#7335=EDGE_LOOP ( 'NONE', ( #17769, #15134, #8661, #6053 ) ) ;
#7346=EDGE_CURVE ( 'NONE', #15544, #3222, #8406, .T. ) ;
#7369=DIRECTION ( 'NONE',  ( -0.000000000000000000, -1.000000000000000000, -0.000000000000000000 ) ) ;
#7377=AXIS2_PLACEMENT_3D ( 'NONE', #17150, #14245, #7200 ) ;
#7378=CIRCLE ( 'NONE', #2291, 8.000000000000000000 ) ;
#7407=EDGE_LOOP ( 'NONE', ( #1362, #18018, #3327, #7490, #12615, #11532 ) ) ;
#7408=LINE ( 'NONE', #13533, #15564 ) ;
#7426=LINE ( 'NONE', #9153, #7102 ) ;
#7447=ORIENTED_EDGE ( 'NONE', *, *, #17815, .T. ) ;
#7466=CARTESIAN_POINT ( 'NONE',  ( -19.00000000000000355, 3.278623949159157558, -2.625000000000002220 ) ) ;
#7490=ORIENTED_EDGE ( 'NONE', *, *, #12482, .F. ) ;
#7560=EDGE_CURVE ( 'NONE', #18392, #530, #7572, .T. ) ;
#7563=ORIENTED_EDGE ( 'NONE', *, *, #11668, .T. ) ;
#7571=EDGE_CURVE ( 'NONE', #4614, #16516, #14460, .T. ) ;
#7572=LINE ( 'NONE', #10692, #17011 ) ;
#7593=DIRECTION ( 'NONE',  ( 1.000000000000000000, 6.419766481290786633E-33, -0.000000000000000000 ) ) ;
#7620=EDGE_LOOP ( 'NONE', ( #13782, #9777, #10149, #6335 ) ) ;
#7621=CARTESIAN_POINT ( 'NONE',  ( -11.00000000000000355, 4.215373648918917304, -3.375000000000002665 ) ) ;
#7669=DIRECTION ( 'NONE',  ( 1.000000000000000000, 6.419766481290786633E-33, -0.000000000000000000 ) ) ;
#7706=AXIS2_PLACEMENT_3D ( 'NONE', #9829, #5101, #11215 ) ;
#7708=VECTOR ( 'NONE', #2628, 1000.000000000000000 ) ;
#7721=CARTESIAN_POINT ( 'NONE',  ( -36.00000000000000000, 4.999999999999999112, -2.000000000000000000 ) ) ;
#7723=VECTOR ( 'NONE', #19277, 1000.000000000000000 ) ;
#7734=CARTESIAN_POINT ( 'NONE',  ( -41.99999999999999289, 4.999999999999998224, -2.000000000000000000 ) ) ;
#7753=ORIENTED_EDGE ( 'NONE', *, *, #18156, .T. ) ;
#7757=EDGE_CURVE ( 'NONE', #14026, #10153, #19253, .T. ) ;
#7779=EDGE_CURVE ( 'NONE', #10940, #6746, #6854, .T. ) ;
#7784=CARTESIAN_POINT ( 'NONE',  ( -11.00000000000000355, -3.278623949159158446, -2.625000000000002220 ) ) ;
#7790=ORIENTED_EDGE ( 'NONE', *, *, #6750, .T. ) ;
#7827=LINE ( 'NONE', #29, #4093 ) ;
#7829=CARTESIAN_POINT ( 'NONE',  ( -36.00000000000000000, -2.311115933264683024E-31, 0.000000000000000000 ) ) ;
#7837=DIRECTION ( 'NONE',  ( -1.000000000000000000, -1.224646799147353207E-16, 0.000000000000000000 ) ) ;
#7842=PRODUCT_CONTEXT ( 'NONE', #8430, 'mechanical' ) ;
#7857=CARTESIAN_POINT ( 'NONE',  ( -11.00000000000000355, 3.278623949159158446, -2.625000000000002220 ) ) ;
#7867=DIRECTION ( 'NONE',  ( 1.000000000000000000, 6.419766481290786633E-33, -0.000000000000000000 ) ) ;
#7869=DIRECTION ( 'NONE',  ( 0.000000000000000000, 1.000000000000000000, 0.000000000000000000 ) ) ;
#7887=CARTESIAN_POINT ( 'NONE',  ( -10.99900000000000233, -7.061101152771736665E-32, 0.000000000000000000 ) ) ;
#7904=CIRCLE ( 'NONE', #18763, 4.400000000000000355 ) ;
#7931=FACE_OUTER_BOUND ( 'NONE', #1907, .T. ) ;
#7949=CIRCLE ( 'NONE', #9569, 6.000000000000000888 ) ;
#7958=DIRECTION ( 'NONE',  ( 1.000000000000000000, 1.224646799147353207E-16, -0.000000000000000000 ) ) ;
#7962=CYLINDRICAL_SURFACE ( 'NONE', #12422, 4.200000000000000178 ) ;
#7997=CIRCLE ( 'NONE', #9614, 4.200000000000000178 ) ;
#8013=DIRECTION ( 'NONE',  ( -7.654042494670960318E-17, 0.6250000000000002220, 0.7806247497997995666 ) ) ;
#8034=DIRECTION ( 'NONE',  ( 1.000000000000000000, 1.224646799147353207E-16, -0.000000000000000000 ) ) ;
#8056=DIRECTION ( 'NONE',  ( -9.559896011775280412E-17, 0.7806247497997995666, -0.6250000000000002220 ) ) ;
#8059=LINE ( 'NONE', #9578, #565 ) ;
#8060=SURFACE_STYLE_FILL_AREA ( #15677 ) ;
#8066=ADVANCED_FACE ( 'NONE', ( #10942, #17048 ), #438, .T. ) ;
#8099=DIRECTION ( 'NONE',  ( 1.000000000000000000, 1.224646799147353207E-16, 0.000000000000000000 ) ) ;
#8118=FACE_OUTER_BOUND ( 'NONE', #3492, .T. ) ;
#8122=ORIENTED_EDGE ( 'NONE', *, *, #6407, .F. ) ;
#8138=DIRECTION ( 'NONE',  ( -1.000000000000000000, -6.419766481290788001E-33, -0.000000000000000000 ) ) ;
#8152=ORIENTED_EDGE ( 'NONE', *, *, #527, .T. ) ;
#8154=CARTESIAN_POINT ( 'NONE',  ( -36.00000000000000000, -5.000000000000000888, -2.000000000000000000 ) ) ;
#8163=CARTESIAN_POINT ( 'NONE',  ( -15.00000000000000355, 0.000000000000000000, 0.000000000000000000 ) ) ;
#8168=ADVANCED_FACE ( 'NONE', ( #9850 ), #2511, .T. ) ;
#8172=DIRECTION ( 'NONE',  ( -1.000000000000000000, -6.419766481290786633E-33, 0.000000000000000000 ) ) ;
#8180=VERTEX_POINT ( 'NONE', #927 ) ;
#8184=DIRECTION ( 'NONE',  ( -1.000000000000000000, -1.224646799147353207E-16, 0.000000000000000000 ) ) ;
#8200=LINE ( 'NONE', #11107, #1244 ) ;
#8225=VERTEX_POINT ( 'NONE', #11922 ) ;
#8267=DIRECTION ( 'NONE',  ( -1.000000000000000000, -6.419766481290786633E-33, 0.000000000000000000 ) ) ;
#8275=DIRECTION ( 'NONE',  ( -1.000000000000000000, 0.000000000000000000, 0.000000000000000000 ) ) ;
#8331=EDGE_CURVE ( 'NONE', #17936, #15544, #9975, .T. ) ;
#8356=EDGE_CURVE ( 'NONE', #17288, #2407, #7378, .T. ) ;
#8360=DIRECTION ( 'NONE',  ( -1.000000000000000000, 0.000000000000000000, 0.000000000000000000 ) ) ;
#8368=CARTESIAN_POINT ( 'NONE',  ( -15.00000000000000355, 4.400000000000000355, 0.000000000000000000 ) ) ;
#8392=AXIS2_PLACEMENT_3D ( 'NONE', #11066, #15870, #8360 ) ;
#8406=LINE ( 'NONE', #9818, #6138 ) ;
#8430=APPLICATION_CONTEXT ( 'automotive_design' ) ;
#8437=DIRECTION ( 'NONE',  ( 1.000000000000000000, 1.224646799147353207E-16, -0.000000000000000000 ) ) ;
#8488=EDGE_LOOP ( 'NONE', ( #1330, #10081, #19024, #14617 ) ) ;
#8498=AXIS2_PLACEMENT_3D ( 'NONE', #2171, #8275, #9894 ) ;
#8508=EDGE_CURVE ( 'NONE', #2009, #5745, #11696, .T. ) ;
#8555=ORIENTED_EDGE ( 'NONE', *, *, #19538, .T. ) ;
#8624=CYLINDRICAL_SURFACE ( 'NONE', #13466, 5.400000000000000355 ) ;
#8628=VECTOR ( 'NONE', #12389, 1000.000000000000000 ) ;
#8653=CARTESIAN_POINT ( 'NONE',  ( -41.99999999999999289, -5.000000000000001776, 2.000000000000000000 ) ) ;
#8661=ORIENTED_EDGE ( 'NONE', *, *, #1414, .T. ) ;
#8668=DIRECTION ( 'NONE',  ( 0.000000000000000000, 0.000000000000000000, 1.000000000000000000 ) ) ;
#8705=FACE_OUTER_BOUND ( 'NONE', #3173, .T. ) ;
#8732=EDGE_CURVE ( 'NONE', #17039, #14026, #784, .T. ) ;
#8778=DIRECTION ( 'NONE',  ( 0.000000000000000000, 1.000000000000000000, 0.000000000000000000 ) ) ;
#8785=( NAMED_UNIT ( * ) PLANE_ANGLE_UNIT ( ) SI_UNIT ( $, .RADIAN. ) );
#8786=CARTESIAN_POINT ( 'NONE',  ( -30.00000000000000000, -8.000000000000000000, 9.797174393178825657E-16 ) ) ;
#8852=EDGE_CURVE ( 'NONE', #8225, #12806, #12854, .T. ) ;
#8862=CIRCLE ( 'NONE', #15255, 4.200000000000000178 ) ;
#8874=FACE_OUTER_BOUND ( 'NONE', #6329, .T. ) ;
#8876=VECTOR ( 'NONE', #7593, 1000.000000000000000 ) ;
#8898=ORIENTED_EDGE ( 'NONE', *, *, #19711, .F. ) ;
#8901=AXIS2_PLACEMENT_3D ( 'NONE', #17771, #19460, #5747 ) ;
#8907=CARTESIAN_POINT ( 'NONE',  ( -30.00000000000000000, -4.200000000000000178, 0.000000000000000000 ) ) ;
#8914=CARTESIAN_POINT ( 'NONE',  ( -41.99999999999999289, 4.399999999999997691, 0.000000000000000000 ) ) ;
#8926=VECTOR ( 'NONE', #6783, 1000.000000000000000 ) ;
#8946=ADVANCED_FACE ( 'NONE', ( #8874 ), #13179, .T. ) ;
#8952=ORIENTED_EDGE ( 'NONE', *, *, #11176, .T. ) ;
#8988=PRODUCT_DEFINITION_CONTEXT ( 'detailed design', #11110, 'design' ) ;
#8989=CARTESIAN_POINT ( 'NONE',  ( -30.00000000000000000, -4.400000000000000355, 5.388445916248354013E-16 ) ) ;
#9042=DIRECTION ( 'NONE',  ( 1.000000000000000000, 1.224646799147353207E-16, -0.000000000000000000 ) ) ;
#9050=AXIS2_PLACEMENT_3D ( 'NONE', #19750, #15058, #5739 ) ;
#9052=DIRECTION ( 'NONE',  ( 0.000000000000000000, 0.000000000000000000, 1.000000000000000000 ) ) ;
#9072=CARTESIAN_POINT ( 'NONE',  ( -19.00000000000000355, 1.224646799147353207E-16, 0.000000000000000000 ) ) ;
#9076=PRODUCT_DEFINITION ( 'UNKNOWN', '', #3478, #8988 ) ;
#9078=COLOUR_RGB ( '', 0.09019608, 0.27058824, 0.51372549) ;
#9087=CARTESIAN_POINT ( 'NONE',  ( -36.00000000000000000, 6.000000000000000888, 0.000000000000000000 ) ) ;
#9153=CARTESIAN_POINT ( 'NONE',  ( -41.99999999999999289, -2.000000000000001776, -5.000000000000000000 ) ) ;
#9172=VERTEX_POINT ( 'NONE', #3758 ) ;
#9178=DIRECTION ( 'NONE',  ( 1.224646799147353207E-16, -1.000000000000000000, 0.000000000000000000 ) ) ;
#9180=CARTESIAN_POINT ( 'NONE',  ( -36.00000000000000000, -6.000000000000000888, 7.347880794884120722E-16 ) ) ;
#9188=CARTESIAN_POINT ( 'NONE',  ( -36.00000000000000000, -2.000000000000000888, 2.000000000000000000 ) ) ;
#9193=AXIS2_PLACEMENT_3D ( 'NONE', #1917, #8013, #14127 ) ;
#9198=EDGE_CURVE ( 'NONE', #17288, #14054, #16375, .T. ) ;
#9200=MANIFOLD_SOLID_BREP ( 'Cut-Extrude1', #18617 ) ;
#9233=ORIENTED_EDGE ( 'NONE', *, *, #12851, .T. ) ;
#9264=VERTEX_POINT ( 'NONE', #952 ) ;
#9334=LINE ( 'NONE', #13834, #14945 ) ;
#9345=DIRECTION ( 'NONE',  ( -1.000000000000000000, -6.419766481290786633E-33, 0.000000000000000000 ) ) ;
#9353=VECTOR ( 'NONE', #8056, 1000.000000000000000 ) ;
#9391=EDGE_CURVE ( 'NONE', #17967, #12806, #140, .T. ) ;
#9399=VERTEX_POINT ( 'NONE', #3137 ) ;
#9434=DIRECTION ( 'NONE',  ( 0.000000000000000000, 1.000000000000000000, 0.000000000000000000 ) ) ;
#9438=CARTESIAN_POINT ( 'NONE',  ( -36.00000000000000000, 1.999999999999999112, 5.000000000000000000 ) ) ;
#9461=CYLINDRICAL_SURFACE ( 'NONE', #6202, 3.000000000000000000 ) ;
#9483=( NAMED_UNIT ( * ) SI_UNIT ( $, .STERADIAN. ) SOLID_ANGLE_UNIT ( ) );
#9492=CARTESIAN_POINT ( 'NONE',  ( -41.99999999999999289, -2.000000000000001776, 2.000000000000000000 ) ) ;
#9522=DIRECTION ( 'NONE',  ( 0.000000000000000000, -3.552713678800500929E-15, 1.000000000000000000 ) ) ;
#9569=AXIS2_PLACEMENT_3D ( 'NONE', #4142, #13148, #4047 ) ;
#9578=CARTESIAN_POINT ( 'NONE',  ( -15.00000000000000355, 3.434748899119117294, -2.750000000000002220 ) ) ;
#9607=DIRECTION ( 'NONE',  ( 1.000000000000000000, 6.419766481290786633E-33, -0.000000000000000000 ) ) ;
#9614=AXIS2_PLACEMENT_3D ( 'NONE', #16421, #11916, #4499 ) ;
#9621=ORIENTED_EDGE ( 'NONE', *, *, #18502, .T. ) ;
#9625=DIRECTION ( 'NONE',  ( -1.000000000000000000, -1.224646799147353207E-16, 0.000000000000000000 ) ) ;
#9647=VERTEX_POINT ( 'NONE', #12399 ) ;
#9675=ORIENTED_EDGE ( 'NONE', *, *, #10431, .T. ) ;
#9686=( LENGTH_UNIT ( ) NAMED_UNIT ( * ) SI_UNIT ( .MILLI., .METRE. ) );
#9702=ADVANCED_FACE ( 'NONE', ( #1588 ), #90, .T. ) ;
#9711=CYLINDRICAL_SURFACE ( 'NONE', #17417, 4.200000000000000178 ) ;
#9777=ORIENTED_EDGE ( 'NONE', *, *, #6631, .T. ) ;
#9778=( LENGTH_UNIT ( ) NAMED_UNIT ( * ) SI_UNIT ( .MILLI., .METRE. ) );
#9808=DIRECTION ( 'NONE',  ( 0.000000000000000000, -1.000000000000000000, 0.000000000000000000 ) ) ;
#9818=CARTESIAN_POINT ( 'NONE',  ( -11.00000000000000355, -5.400000000000001243, 0.000000000000000000 ) ) ;
#9828=FACE_OUTER_BOUND ( 'NONE', #14495, .T. ) ;
#9829=CARTESIAN_POINT ( 'NONE',  ( -30.00000000000000000, -1.925929944387235853E-31, 0.000000000000000000 ) ) ;
#9830=DIRECTION ( 'NONE',  ( 1.000000000000000000, 6.419766481290786633E-33, -0.000000000000000000 ) ) ;
#9833=DIRECTION ( 'NONE',  ( 0.000000000000000000, 0.000000000000000000, 1.000000000000000000 ) ) ;
#9840=ORIENTED_EDGE ( 'NONE', *, *, #6094, .F. ) ;
#9850=FACE_OUTER_BOUND ( 'NONE', #14936, .T. ) ;
#9851=DIRECTION ( 'NONE',  ( 9.559896011775280412E-17, 0.7806247497997995666, -0.6250000000000001110 ) ) ;
#9894=DIRECTION ( 'NONE',  ( 0.000000000000000000, 0.000000000000000000, 1.000000000000000000 ) ) ;
#9901=FACE_OUTER_BOUND ( 'NONE', #6031, .T. ) ;
#9922=ADVANCED_FACE ( 'NONE', ( #5664 ), #13184, .F. ) ;
#9929=DIRECTION ( 'NONE',  ( 0.000000000000000000, 1.000000000000000000, 0.000000000000000000 ) ) ;
#9945=DIRECTION ( 'NONE',  ( -7.861946472586228936E-49, 1.224646799147353207E-16, 1.000000000000000000 ) ) ;
#9961=ORIENTED_EDGE ( 'NONE', *, *, #15150, .F. ) ;
#9969=DIRECTION ( 'NONE',  ( -1.000000000000000000, 1.224646799147353207E-16, 0.000000000000000000 ) ) ;
#9975=CIRCLE ( 'NONE', #13789, 5.400000000000000355 ) ;
#9997=CARTESIAN_POINT ( 'NONE',  ( -19.00000000000000355, 3.278623949159157558, -2.625000000000002220 ) ) ;
#10003=AXIS2_PLACEMENT_3D ( 'NONE', #7829, #9345, #11141 ) ;
#10008=CARTESIAN_POINT ( 'NONE',  ( -41.99999999999999289, -2.000000000000001776, -5.000000000000000000 ) ) ;
#10023=CARTESIAN_POINT ( 'NONE',  ( -36.00000000000000000, -2.311115933264683024E-31, 0.000000000000000000 ) ) ;
#10024=AXIS2_PLACEMENT_3D ( 'NONE', #17244, #18741, #240 ) ;
#10044=CARTESIAN_POINT ( 'NONE',  ( -41.99999999999999289, 4.999999999999998224, 5.000000000000000000 ) ) ;
#10055=AXIS2_PLACEMENT_3D ( 'NONE', #15992, #2282, #6059 ) ;
#10067=DIRECTION ( 'NONE',  ( -1.000000000000000000, 1.224646799147353207E-16, 0.000000000000000000 ) ) ;
#10076=LINE ( 'NONE', #8368, #10312 ) ;
#10081=ORIENTED_EDGE ( 'NONE', *, *, #12844, .F. ) ;
#10107=ORIENTED_EDGE ( 'NONE', *, *, #13571, .T. ) ;
#10118=ORIENTED_EDGE ( 'NONE', *, *, #8356, .T. ) ;
#10149=ORIENTED_EDGE ( 'NONE', *, *, #2944, .T. ) ;
#10153=VERTEX_POINT ( 'NONE', #15044 ) ;
#10164=CIRCLE ( 'NONE', #7259, 3.000000000000000000 ) ;
#10216=ORIENTED_EDGE ( 'NONE', *, *, #17176, .F. ) ;
#10240=CIRCLE ( 'NONE', #18540, 3.000000000000000000 ) ;
#10254=DIRECTION ( 'NONE',  ( -1.000000000000000000, -1.224646799147353207E-16, 0.000000000000000000 ) ) ;
#10256=DIRECTION ( 'NONE',  ( 0.000000000000000000, 1.000000000000000000, 0.000000000000000000 ) ) ;
#10261=( NAMED_UNIT ( * ) SI_UNIT ( $, .STERADIAN. ) SOLID_ANGLE_UNIT ( ) );
#10283=CARTESIAN_POINT ( 'NONE',  ( -41.99999999999999289, 1.999999999999998224, 2.000000000000000000 ) ) ;
#10297=CARTESIAN_POINT ( 'NONE',  ( -15.00000000000000355, -5.400000000000000355, 0.000000000000000000 ) ) ;
#10304=EDGE_CURVE ( 'NONE', #9647, #14916, #12967, .T. ) ;
#10312=VECTOR ( 'NONE', #5356, 1000.000000000000000 ) ;
#10349=CARTESIAN_POINT ( 'NONE',  ( -30.00000000000000000, -1.925929944387235853E-31, 0.000000000000000000 ) ) ;
#10363=PLANE ( 'NONE',  #14423 ) ;
#10389=CARTESIAN_POINT ( 'NONE',  ( -36.00000000000000000, 1.224646799147351975E-16, 0.000000000000000000 ) ) ;
#10409=AXIS2_PLACEMENT_3D ( 'NONE', #18450, #6229, #15652 ) ;
#10428=EDGE_CURVE ( 'NONE', #3802, #11052, #16478, .T. ) ;
#10431=EDGE_CURVE ( 'NONE', #12806, #5646, #18745, .T. ) ;
#10436=CIRCLE ( 'NONE', #4688, 4.400000000000000355 ) ;
#10455=ADVANCED_FACE ( 'NONE', ( #5131 ), #14250, .F. ) ;
#10488=ORIENTED_EDGE ( 'NONE', *, *, #18616, .T. ) ;
#10511=CARTESIAN_POINT ( 'NONE',  ( -15.00000000000000355, 8.000000000000000000, 0.000000000000000000 ) ) ;
#10570=VECTOR ( 'NONE', #702, 1000.000000000000000 ) ;
#10598=ORIENTED_EDGE ( 'NONE', *, *, #19004, .F. ) ;
#10622=CARTESIAN_POINT ( 'NONE',  ( -36.00000000000000000, -4.200000000000000178, 0.000000000000000000 ) ) ;
#10626=AXIS2_PLACEMENT_3D ( 'NONE', #12187, #1685, #7869 ) ;
#10638=ORIENTED_EDGE ( 'NONE', *, *, #777, .F. ) ;
#10652=VECTOR ( 'NONE', #6697, 1000.000000000000000 ) ;
#10673=DIRECTION ( 'NONE',  ( -1.000000000000000000, 1.224646799147353207E-16, 0.000000000000000000 ) ) ;
#10692=CARTESIAN_POINT ( 'NONE',  ( -15.00000000000000355, 4.874999999999997335, -3.903123748998999609 ) ) ;
#10719=ORIENTED_EDGE ( 'NONE', *, *, #18156, .F. ) ;
#10777=ORIENTED_EDGE ( 'NONE', *, *, #8732, .T. ) ;
#10779=DIRECTION ( 'NONE',  ( 0.000000000000000000, 1.776356839400250465E-15, 1.000000000000000000 ) ) ;
#10784=DIRECTION ( 'NONE',  ( 0.000000000000000000, -1.000000000000000000, 0.000000000000000000 ) ) ;
#10808=ORIENTED_EDGE ( 'NONE', *, *, #8852, .F. ) ;
#10818=ORIENTED_EDGE ( 'NONE', *, *, #13741, .T. ) ;
#10848=CARTESIAN_POINT ( 'NONE',  ( -19.00000000000000355, 3.434748899119118626, 2.750000000000001776 ) ) ;
#10905=DIRECTION ( 'NONE',  ( 0.000000000000000000, -8.881784197001252323E-16, 1.000000000000000000 ) ) ;
#10906=AXIS2_PLACEMENT_3D ( 'NONE', #12841, #337, #3440 ) ;
#10926=ADVANCED_FACE ( 'NONE', ( #5501, #8705 ), #2891, .T. ) ;
#10930=CARTESIAN_POINT ( 'NONE',  ( -11.00000000000000355, -5.400000000000001243, 0.000000000000000000 ) ) ;
#10937=AXIS2_PLACEMENT_3D ( 'NONE', #3981, #885, #2468 ) ;
#10940=VERTEX_POINT ( 'NONE', #16414 ) ;
#10942=FACE_BOUND ( 'NONE', #19335, .T. ) ;
#10953=VECTOR ( 'NONE', #15784, 1000.000000000000114 ) ;
#10965=CARTESIAN_POINT ( 'NONE',  ( -19.00000000000000355, -4.400000000000000355, 5.388445916248354013E-16 ) ) ;
#10970=VECTOR ( 'NONE', #11632, 1000.000000000000000 ) ;
#10977=CARTESIAN_POINT ( 'NONE',  ( -15.00000000000000355, 3.434748899119118182, -2.750000000000002665 ) ) ;
#10991=VERTEX_POINT ( 'NONE', #4400 ) ;
#11004=AXIS2_PLACEMENT_3D ( 'NONE', #11451, #2525, #7018 ) ;
#11011=AXIS2_PLACEMENT_3D ( 'NONE', #18918, #3322, #9434 ) ;
#11029=ORIENTED_EDGE ( 'NONE', *, *, #3900, .T. ) ;
#11037=VECTOR ( 'NONE', #13679, 1000.000000000000000 ) ;
#11052=VERTEX_POINT ( 'NONE', #1109 ) ;
#11066=CARTESIAN_POINT ( 'NONE',  ( -22.50000000000000711, -21.04737509655562988, 0.000000000000000000 ) ) ;
#11107=CARTESIAN_POINT ( 'NONE',  ( -11.00000000000000355, 4.215373648918917304, -3.375000000000002665 ) ) ;
#11110=APPLICATION_CONTEXT ( 'automotive_design' ) ;
#11114=DIRECTION ( 'NONE',  ( 0.000000000000000000, 1.000000000000000000, 0.000000000000000000 ) ) ;
#11141=DIRECTION ( 'NONE',  ( 6.419766481290786633E-33, -1.000000000000000000, 0.000000000000000000 ) ) ;
#11172=LINE ( 'NONE', #359, #5511 ) ;
#11176=EDGE_CURVE ( 'NONE', #16982, #11206, #10436, .T. ) ;
#11182=DIRECTION ( 'NONE',  ( 0.000000000000000000, 0.000000000000000000, 1.000000000000000000 ) ) ;
#11197=FACE_OUTER_BOUND ( 'NONE', #7620, .T. ) ;
#11206=VERTEX_POINT ( 'NONE', #17691 ) ;
#11215=DIRECTION ( 'NONE',  ( 0.000000000000000000, -1.000000000000000000, 0.000000000000000000 ) ) ;
#11244=CARTESIAN_POINT ( 'NONE',  ( -15.00000000000000355, 1.224646799147353454E-16, 0.000000000000000000 ) ) ;
#11245=CARTESIAN_POINT ( 'NONE',  ( -11.00000000000000355, 4.898587196589412829E-16, 0.000000000000000000 ) ) ;
#11262=PRESENTATION_STYLE_ASSIGNMENT (( #6840 ) ) ;
#11264=CIRCLE ( 'NONE', #5805, 4.400000000000000355 ) ;
#11265=ORIENTED_EDGE ( 'NONE', *, *, #16897, .F. ) ;
#11283=DIRECTION ( 'NONE',  ( -1.000000000000000000, 0.000000000000000000, 0.000000000000000000 ) ) ;
#11285=PLANE ( 'NONE',  #8498 ) ;
#11307=CARTESIAN_POINT ( 'NONE',  ( -36.00000000000000000, -5.000000000000001776, 5.000000000000000000 ) ) ;
#11327=STYLED_ITEM ( 'NONE', ( #18672 ), #3271 ) ;
#11331=FACE_OUTER_BOUND ( 'NONE', #12748, .T. ) ;
#11335=DIRECTION ( 'NONE',  ( -1.000000000000000000, -6.419766481290786633E-33, 0.000000000000000000 ) ) ;
#11344=EDGE_LOOP ( 'NONE', ( #14909, #18337, #1902, #15481 ) ) ;
#11347=DIRECTION ( 'NONE',  ( -1.000000000000000000, -6.419766481290786633E-33, 0.000000000000000000 ) ) ;
#11401=UNCERTAINTY_MEASURE_WITH_UNIT (LENGTH_MEASURE( 1.000000000000000082E-05 ), #9686, 'distance_accuracy_value', 'NONE');
#11418=CARTESIAN_POINT ( 'NONE',  ( -15.00000000000000355, 1.224646799147353454E-16, 0.000000000000000000 ) ) ;
#11451=CARTESIAN_POINT ( 'NONE',  ( -15.00000000000000355, 1.224646799147353454E-16, 0.000000000000000000 ) ) ;
#11453=EDGE_CURVE ( 'NONE', #8180, #9399, #13283, .T. ) ;
#11488=LINE ( 'NONE', #9997, #7723 ) ;
#11503=VERTEX_POINT ( 'NONE', #12383 ) ;
#11526=DIRECTION ( 'NONE',  ( 0.000000000000000000, -1.000000000000000000, 1.224646799147353207E-16 ) ) ;
#11530=EDGE_CURVE ( 'NONE', #3019, #8180, #8862, .T. ) ;
#11532=ORIENTED_EDGE ( 'NONE', *, *, #2002, .F. ) ;
#11537=ORIENTED_EDGE ( 'NONE', *, *, #13571, .F. ) ;
#11545=CARTESIAN_POINT ( 'NONE',  ( -11.00000000000000355, -3.278623949159158446, -2.625000000000002220 ) ) ;
#11569=ORIENTED_EDGE ( 'NONE', *, *, #17176, .T. ) ;
#11574=VECTOR ( 'NONE', #5073, 1000.000000000000000 ) ;
#11578=LINE ( 'NONE', #18080, #6259 ) ;
#11587=EDGE_CURVE ( 'NONE', #14330, #4430, #15578, .T. ) ;
#11599=VERTEX_POINT ( 'NONE', #10977 ) ;
#11602=ORIENTED_EDGE ( 'NONE', *, *, #14642, .T. ) ;
#11619=EDGE_CURVE ( 'NONE', #4430, #12789, #6165, .T. ) ;
#11623=ORIENTED_EDGE ( 'NONE', *, *, #19029, .F. ) ;
#11629=( GEOMETRIC_REPRESENTATION_CONTEXT ( 3 ) GLOBAL_UNCERTAINTY_ASSIGNED_CONTEXT ( ( #11401 ) ) GLOBAL_UNIT_ASSIGNED_CONTEXT ( ( #9686, #3170, #9483 ) ) REPRESENTATION_CONTEXT ( 'NONE', 'WORKASPACE' ) );
#11632=DIRECTION ( 'NONE',  ( 0.000000000000000000, 0.000000000000000000, -1.000000000000000000 ) ) ;
#11643=PLANE ( 'NONE',  #16668 ) ;
#11668=EDGE_CURVE ( 'NONE', #11599, #4605, #8059, .T. ) ;
#11677=DIRECTION ( 'NONE',  ( 1.000000000000000000, 6.419766481290786633E-33, -0.000000000000000000 ) ) ;
#11696=LINE ( 'NONE', #16210, #19225 ) ;
#11718=CYLINDRICAL_SURFACE ( 'NONE', #16522, 4.400000000000000355 ) ;
#11728=DIRECTION ( 'NONE',  ( -1.000000000000000000, 1.224646799147353207E-16, 0.000000000000000000 ) ) ;
#11739=ORIENTED_EDGE ( 'NONE', *, *, #2889, .T. ) ;
#11748=CYLINDRICAL_SURFACE ( 'NONE', #4078, 6.000000000000000888 ) ;
#11752=VERTEX_POINT ( 'NONE', #14275 ) ;
#11780=EDGE_CURVE ( 'NONE', #2009, #3616, #12375, .T. ) ;
#11821=CARTESIAN_POINT ( 'NONE',  ( -11.00000000000000355, -4.215373648918918192, 3.375000000000000888 ) ) ;
#11833=ORIENTED_EDGE ( 'NONE', *, *, #7779, .T. ) ;
#11835=ORIENTED_EDGE ( 'NONE', *, *, #5299, .T. ) ;
#11842=CYLINDRICAL_SURFACE ( 'NONE', #14929, 4.200000000000000178 ) ;
#11850=CARTESIAN_POINT ( 'NONE',  ( -11.00000000000000355, 4.215373648918918192, 3.375000000000000888 ) ) ;
#11855=CARTESIAN_POINT ( 'NONE',  ( -30.00000000000000000, -6.000000000000000888, 7.347880794884120722E-16 ) ) ;
#11864=FACE_OUTER_BOUND ( 'NONE', #7407, .T. ) ;
#11873=AXIS2_PLACEMENT_3D ( 'NONE', #18713, #617, #14116 ) ;
#11885=CARTESIAN_POINT ( 'NONE',  ( -19.00000000000000355, -3.434748899119117294, -2.750000000000002220 ) ) ;
#11893=EDGE_CURVE ( 'NONE', #10940, #18392, #7408, .T. ) ;
#11897=DIRECTION ( 'NONE',  ( 0.000000000000000000, 0.000000000000000000, 1.000000000000000000 ) ) ;
#11912=FACE_OUTER_BOUND ( 'NONE', #957, .T. ) ;
#11916=DIRECTION ( 'NONE',  ( -1.000000000000000000, 1.224646799147353207E-16, 0.000000000000000000 ) ) ;
#11922=CARTESIAN_POINT ( 'NONE',  ( -41.99999999999999289, 1.999999999999998224, 5.000000000000000000 ) ) ;
#11947=MECHANICAL_DESIGN_GEOMETRIC_PRESENTATION_REPRESENTATION('',(#11327),#11629);
#11950=VERTEX_POINT ( 'NONE', #9438 ) ;
#11954=LINE ( 'NONE', #16560, #14152 ) ;
#11966=PLANE ( 'NONE',  #8901 ) ;
#11974=CARTESIAN_POINT ( 'NONE',  ( -22.50000000000000711, 0.000000000000000000, 0.000000000000000000 ) ) ;
#11980=EDGE_CURVE ( 'NONE', #3279, #123, #9334, .T. ) ;
#12028=ADVANCED_FACE ( 'NONE', ( #4927 ), #6603, .F. ) ;
#12042=ORIENTED_EDGE ( 'NONE', *, *, #18823, .F. ) ;
#12070=VERTEX_POINT ( 'NONE', #14329 ) ;
#12077=SHAPE_REPRESENTATION ( 'brake cone', ( #16724 ), #3651 ) ;
#12081=AXIS2_PLACEMENT_3D ( 'NONE', #17825, #8437, #19315 ) ;
#12094=CIRCLE ( 'NONE', #16565, 6.000000000000000888 ) ;
#12101=VERTEX_POINT ( 'NONE', #5411 ) ;
#12147=CARTESIAN_POINT ( 'NONE',  ( -15.00000000000000355, -3.434748899119118182, -2.750000000000002665 ) ) ;
#12154=FACE_OUTER_BOUND ( 'NONE', #6381, .T. ) ;
#12159=DIRECTION ( 'NONE',  ( 1.000000000000000000, 1.224646799147353207E-16, 0.000000000000000000 ) ) ;
#12176=FACE_OUTER_BOUND ( 'NONE', #3509, .T. ) ;
#12181=CARTESIAN_POINT ( 'NONE',  ( -11.00000000000000355, -4.200000000000001066, 0.000000000000000000 ) ) ;
#12184=FACE_OUTER_BOUND ( 'NONE', #19775, .T. ) ;
#12187=CARTESIAN_POINT ( 'NONE',  ( -15.00000000000000355, 0.000000000000000000, 0.000000000000000000 ) ) ;
#12191=EDGE_CURVE ( 'NONE', #11206, #16982, #7904, .T. ) ;
#12194=AXIS2_PLACEMENT_3D ( 'NONE', #7313, #14942, #4525 ) ;
#12221=ORIENTED_EDGE ( 'NONE', *, *, #18616, .F. ) ;
#12251=EDGE_CURVE ( 'NONE', #2365, #9647, #5993, .T. ) ;
#12325=CARTESIAN_POINT ( 'NONE',  ( -11.00000000000000355, -4.898587196589412829E-16, 0.000000000000000000 ) ) ;
#12375=CIRCLE ( 'NONE', #3753, 4.200000000000000178 ) ;
#12383=CARTESIAN_POINT ( 'NONE',  ( -11.00000000000000355, 4.215373648918918192, 3.375000000000000888 ) ) ;
#12389=DIRECTION ( 'NONE',  ( 1.000000000000000000, 6.419766481290786633E-33, -0.000000000000000000 ) ) ;
#12399=CARTESIAN_POINT ( 'NONE',  ( -30.00000000000000000, 6.000000000000000888, 0.000000000000000000 ) ) ;
#12403=DIRECTION ( 'NONE',  ( -5.011428603230760289E-33, 0.7806247497997995666, 0.6250000000000001110 ) ) ;
#12412=CARTESIAN_POINT ( 'NONE',  ( -11.00000000000000355, -4.898587196589412829E-16, 0.000000000000000000 ) ) ;
#12422=AXIS2_PLACEMENT_3D ( 'NONE', #18480, #6169, #10784 ) ;
#12457=DIRECTION ( 'NONE',  ( 1.000000000000000000, 1.224646799147353207E-16, 0.000000000000000000 ) ) ;
#12475=CARTESIAN_POINT ( 'NONE',  ( -15.00000000000000355, 4.874999999999998224, 3.903123748998998721 ) ) ;
#12482=EDGE_CURVE ( 'NONE', #15544, #11752, #1860, .T. ) ;
#12486=EDGE_CURVE ( 'NONE', #13382, #10991, #10164, .T. ) ;
#12503=CARTESIAN_POINT ( 'NONE',  ( -22.50000000000000711, 0.000000000000000000, 0.000000000000000000 ) ) ;
#12555=CIRCLE ( 'NONE', #6450, 4.400000000000000355 ) ;
#12571=VERTEX_POINT ( 'NONE', #13002 ) ;
#12584=ORIENTED_EDGE ( 'NONE', *, *, #5299, .F. ) ;
#12586=CARTESIAN_POINT ( 'NONE',  ( -15.00000000000000355, 0.000000000000000000, 0.000000000000000000 ) ) ;
#12615=ORIENTED_EDGE ( 'NONE', *, *, #8331, .F. ) ;
#12638=DIRECTION ( 'NONE',  ( 0.000000000000000000, -1.000000000000000000, 0.000000000000000000 ) ) ;
#12664=CARTESIAN_POINT ( 'NONE',  ( -19.00000000000000355, 1.224646799147353207E-16, 0.000000000000000000 ) ) ;
#12673=DIRECTION ( 'NONE',  ( 1.000000000000000000, 0.000000000000000000, -0.000000000000000000 ) ) ;
#12681=EDGE_LOOP ( 'NONE', ( #19466, #12221, #19382, #6139, #8152, #9961, #166, #6549, #579 ) ) ;
#12689=VECTOR ( 'NONE', #1083, 1000.000000000000000 ) ;
#12691=DIRECTION ( 'NONE',  ( 0.000000000000000000, 0.7806247497997995666, 0.6250000000000002220 ) ) ;
#12694=CARTESIAN_POINT ( 'NONE',  ( -41.99999999999999289, 4.999999999999998224, -2.000000000000000000 ) ) ;
#12696=AXIS2_PLACEMENT_3D ( 'NONE', #3416, #9625, #12819 ) ;
#12710=VERTEX_POINT ( 'NONE', #7466 ) ;
#12737=AXIS2_PLACEMENT_3D ( 'NONE', #3566, #8172, #5268 ) ;
#12748=EDGE_LOOP ( 'NONE', ( #11623, #3572, #655, #2871 ) ) ;
#12767=FILL_AREA_STYLE_COLOUR ( '', #13820 ) ;
#12789=VERTEX_POINT ( 'NONE', #11885 ) ;
#12806=VERTEX_POINT ( 'NONE', #15488 ) ;
#12819=DIRECTION ( 'NONE',  ( 0.000000000000000000, 0.000000000000000000, 1.000000000000000000 ) ) ;
#12838=ORIENTED_EDGE ( 'NONE', *, *, #19266, .T. ) ;
#12840=FACE_OUTER_BOUND ( 'NONE', #17843, .T. ) ;
#12841=CARTESIAN_POINT ( 'NONE',  ( -15.00000000000000355, 1.224646799147353454E-16, 0.000000000000000000 ) ) ;
#12844=EDGE_CURVE ( 'NONE', #12070, #13382, #1679, .T. ) ;
#12851=EDGE_CURVE ( 'NONE', #12571, #17039, #3142, .T. ) ;
#12854=CIRCLE ( 'NONE', #16055, 3.000000000000000000 ) ;
#12900=AXIS2_PLACEMENT_3D ( 'NONE', #6892, #9830, #14713 ) ;
#12911=ADVANCED_FACE ( 'NONE', ( #12184 ), #7962, .F. ) ;
#12930=EDGE_CURVE ( 'NONE', #3019, #12710, #178, .T. ) ;
#12934=CARTESIAN_POINT ( 'NONE',  ( -30.00000000000000000, 4.200000000000000178, 5.143516556418882928E-16 ) ) ;
#12956=DIRECTION ( 'NONE',  ( 0.000000000000000000, -1.000000000000000000, 0.000000000000000000 ) ) ;
#12967=CIRCLE ( 'NONE', #18075, 6.000000000000000888 ) ;
#12982=CARTESIAN_POINT ( 'NONE',  ( -19.00000000000000355, -4.215373648918917304, 3.375000000000000888 ) ) ;
#12985=ORIENTED_EDGE ( 'NONE', *, *, #3458, .T. ) ;
#13002=CARTESIAN_POINT ( 'NONE',  ( -36.00000000000000000, -2.000000000000000888, 5.000000000000000000 ) ) ;
#13010=EDGE_CURVE ( 'NONE', #14916, #9647, #19433, .T. ) ;
#13020=CARTESIAN_POINT ( 'NONE',  ( -11.00000000000000355, -3.278623949159159778, 2.625000000000000888 ) ) ;
#13051=DIRECTION ( 'NONE',  ( 6.419766481290786633E-33, -1.000000000000000000, 0.000000000000000000 ) ) ;
#13054=LINE ( 'NONE', #1040, #7708 ) ;
#13060=ORIENTED_EDGE ( 'NONE', *, *, #15430, .T. ) ;
#13073=ORIENTED_EDGE ( 'NONE', *, *, #1414, .F. ) ;
#13108=ADVANCED_FACE ( 'NONE', ( #11864 ), #11966, .F. ) ;
#13123=DIRECTION ( 'NONE',  ( 0.000000000000000000, 0.000000000000000000, -1.000000000000000000 ) ) ;
#13148=DIRECTION ( 'NONE',  ( -1.000000000000000000, -6.419766481290786633E-33, 0.000000000000000000 ) ) ;
#13158=ORIENTED_EDGE ( 'NONE', *, *, #11668, .F. ) ;
#13179=TOROIDAL_SURFACE ( 'NONE', #7077, -21.04737509655562988, 30.00000000000000355 ) ;
#13184=CYLINDRICAL_SURFACE ( 'NONE', #4004, 4.400000000000000355 ) ;
#13224=PLANE ( 'NONE',  #15344 ) ;
#13235=EDGE_CURVE ( 'NONE', #12789, #4071, #14653, .T. ) ;
#13283=LINE ( 'NONE', #16291, #12689 ) ;
#13302=ORIENTED_EDGE ( 'NONE', *, *, #1295, .F. ) ;
#13326=ORIENTED_EDGE ( 'NONE', *, *, #2961, .F. ) ;
#13333=ORIENTED_EDGE ( 'NONE', *, *, #6204, .F. ) ;
#13348=DIRECTION ( 'NONE',  ( 0.000000000000000000, -1.000000000000000000, 0.000000000000000000 ) ) ;
#13359=EDGE_CURVE ( 'NONE', #6326, #4605, #4756, .T. ) ;
#13380=( NAMED_UNIT ( * ) SI_UNIT ( $, .STERADIAN. ) SOLID_ANGLE_UNIT ( ) );
#13382=VERTEX_POINT ( 'NONE', #8154 ) ;
#13419=ORIENTED_EDGE ( 'NONE', *, *, #4199, .F. ) ;
#13424=AXIS2_PLACEMENT_3D ( 'NONE', #12503, #15510, #17203 ) ;
#13444=DIRECTION ( 'NONE',  ( -6.419766481290786633E-33, 1.000000000000000000, 0.000000000000000000 ) ) ;
#13466=AXIS2_PLACEMENT_3D ( 'NONE', #5612, #11728, #15128 ) ;
#13503=DIRECTION ( 'NONE',  ( -6.419766481290786633E-33, 1.000000000000000000, 0.000000000000000000 ) ) ;
#13524=DIRECTION ( 'NONE',  ( 9.559896011775280412E-17, -0.7806247497997995666, -0.6250000000000001110 ) ) ;
#13533=CARTESIAN_POINT ( 'NONE',  ( -15.00000000000000355, -3.434748899119118626, 2.750000000000001332 ) ) ;
#13570=ORIENTED_EDGE ( 'NONE', *, *, #11587, .T. ) ;
#13571=EDGE_CURVE ( 'NONE', #2365, #9172, #7949, .T. ) ;
#13594=EDGE_CURVE ( 'NONE', #17943, #6326, #7291, .T. ) ;
#13669=ORIENTED_EDGE ( 'NONE', *, *, #4824, .T. ) ;
#13679=DIRECTION ( 'NONE',  ( 1.000000000000000000, 6.419766481290786633E-33, -0.000000000000000000 ) ) ;
#13707=ORIENTED_EDGE ( 'NONE', *, *, #11530, .T. ) ;
#13720=LINE ( 'NONE', #5907, #2122 ) ;
#13741=EDGE_CURVE ( 'NONE', #16293, #16516, #8200, .T. ) ;
#13745=DIRECTION ( 'NONE',  ( -0.000000000000000000, -0.000000000000000000, 1.000000000000000000 ) ) ;
#13753=DIRECTION ( 'NONE',  ( 0.000000000000000000, -1.000000000000000000, 0.000000000000000000 ) ) ;
#13762=ORIENTED_EDGE ( 'NONE', *, *, #6094, .T. ) ;
#13772=CIRCLE ( 'NONE', #10906, 8.000000000000000000 ) ;
#13776=ORIENTED_EDGE ( 'NONE', *, *, #13594, .F. ) ;
#13779=DIRECTION ( 'NONE',  ( -5.011428603230760289E-33, 0.7806247497997995666, 0.6250000000000002220 ) ) ;
#13782=ORIENTED_EDGE ( 'NONE', *, *, #11780, .T. ) ;
#13783=DIRECTION ( 'NONE',  ( 0.000000000000000000, -1.000000000000000000, 0.000000000000000000 ) ) ;
#13787=AXIS2_PLACEMENT_3D ( 'NONE', #6033, #13947, #15454 ) ;
#13789=AXIS2_PLACEMENT_3D ( 'NONE', #12325, #1716, #9522 ) ;
#13795=EDGE_CURVE ( 'NONE', #17039, #13382, #5391, .T. ) ;
#13810=CARTESIAN_POINT ( 'NONE',  ( -15.00000000000000355, 4.400000000000000355, 0.000000000000000000 ) ) ;
#13820=COLOUR_RGB ( '', 0.09019608, 0.27058824, 0.51372549) ;
#13834=CARTESIAN_POINT ( 'NONE',  ( -41.99999999999999289, -5.000000000000001776, -5.000000000000000000 ) ) ;
#13838=CARTESIAN_POINT ( 'NONE',  ( -36.00000000000000000, -2.311115933264683024E-31, 0.000000000000000000 ) ) ;
#13888=LINE ( 'NONE', #6265, #8628 ) ;
#13889=DIRECTION ( 'NONE',  ( 5.011428603230760289E-33, -0.7806247497997995666, 0.6250000000000001110 ) ) ;
#13913=ORIENTED_EDGE ( 'NONE', *, *, #12482, .T. ) ;
#13916=CARTESIAN_POINT ( 'NONE',  ( -15.00000000000000355, -4.400000000000000355, 5.388445916248354013E-16 ) ) ;
#13924=ADVANCED_FACE ( 'NONE', ( #14167 ), #470, .T. ) ;
#13937=VECTOR ( 'NONE', #14639, 1000.000000000000000 ) ;
#13947=DIRECTION ( 'NONE',  ( -1.000000000000000000, 1.224646799147353207E-16, 0.000000000000000000 ) ) ;
#13958=CARTESIAN_POINT ( 'NONE',  ( -41.99999999999999289, 1.999999999999997335, -5.000000000000000000 ) ) ;
#13966=ORIENTED_EDGE ( 'NONE', *, *, #4561, .T. ) ;
#14007=EDGE_LOOP ( 'NONE', ( #6984, #4330, #13073, #10818 ) ) ;
#14012=FACE_OUTER_BOUND ( 'NONE', #8488, .T. ) ;
#14022=FACE_OUTER_BOUND ( 'NONE', #6843, .T. ) ;
#14026=VERTEX_POINT ( 'NONE', #8653 ) ;
#14054=VERTEX_POINT ( 'NONE', #5258 ) ;
#14075=DIRECTION ( 'NONE',  ( 1.000000000000000000, 1.224646799147353207E-16, 0.000000000000000000 ) ) ;
#14087=CARTESIAN_POINT ( 'NONE',  ( -11.00000000000000355, -3.278623949159158446, -2.625000000000002220 ) ) ;
#14106=FACE_OUTER_BOUND ( 'NONE', #17802, .T. ) ;
#14116=DIRECTION ( 'NONE',  ( 0.000000000000000000, 1.000000000000000000, 0.000000000000000000 ) ) ;
#14124=CARTESIAN_POINT ( 'NONE',  ( -11.00000000000000355, -4.215373648918918192, 3.375000000000000888 ) ) ;
#14127=DIRECTION ( 'NONE',  ( 0.000000000000000000, -0.7806247497997995666, 0.6250000000000002220 ) ) ;
#14147=DIRECTION ( 'NONE',  ( 1.000000000000000000, 1.224646799147353207E-16, -0.000000000000000000 ) ) ;
#14150=FACE_OUTER_BOUND ( 'NONE', #5421, .T. ) ;
#14152=VECTOR ( 'NONE', #6225, 1000.000000000000000 ) ;
#14167=FACE_OUTER_BOUND ( 'NONE', #4025, .T. ) ;
#14173=SURFACE_SIDE_STYLE ('',( #8060 ) ) ;
#14223=CARTESIAN_POINT ( 'NONE',  ( -15.00000000000000355, 3.434748899119118626, 2.750000000000001332 ) ) ;
#14227=PLANE ( 'NONE',  #1921 ) ;
#14245=DIRECTION ( 'NONE',  ( -1.000000000000000000, -6.419766481290786633E-33, 0.000000000000000000 ) ) ;
#14250=PLANE ( 'NONE',  #2413 ) ;
#14252=AXIS2_PLACEMENT_3D ( 'NONE', #9072, #10673, #19563 ) ;
#14257=DIRECTION ( 'NONE',  ( -1.000000000000000000, -6.419766481290786633E-33, 0.000000000000000000 ) ) ;
#14275=CARTESIAN_POINT ( 'NONE',  ( -11.00000000000000355, -4.215373648918918192, 3.375000000000000888 ) ) ;
#14277=AXIS2_PLACEMENT_3D ( 'NONE', #19489, #5778, #11897 ) ;
#14293=CARTESIAN_POINT ( 'NONE',  ( -15.00000000000000355, 4.874999999999998224, 3.903123748998999165 ) ) ;
#14317=ADVANCED_FACE ( 'NONE', ( #5130 ), #16240, .F. ) ;
#14329=CARTESIAN_POINT ( 'NONE',  ( -41.99999999999999289, -5.000000000000001776, -2.000000000000000000 ) ) ;
#14330=VERTEX_POINT ( 'NONE', #3637 ) ;
#14340=FACE_BOUND ( 'NONE', #6219, .T. ) ;
#14350=ORIENTED_EDGE ( 'NONE', *, *, #17815, .F. ) ;
#14354=LINE ( 'NONE', #11545, #6458 ) ;
#14368=EDGE_LOOP ( 'NONE', ( #10107, #17118 ) ) ;
#14378=ORIENTED_EDGE ( 'NONE', *, *, #5496, .F. ) ;
#14400=CARTESIAN_POINT ( 'NONE',  ( -30.00000000000000000, 1.224646799147352468E-16, 0.000000000000000000 ) ) ;
#14423=AXIS2_PLACEMENT_3D ( 'NONE', #11850, #17960, #6863 ) ;
#14460=CIRCLE ( 'NONE', #10626, 5.400000000000000355 ) ;
#14474=MECHANICAL_DESIGN_GEOMETRIC_PRESENTATION_REPRESENTATION('',(#18930),#6217);
#14493=VECTOR ( 'NONE', #13524, 1000.000000000000114 ) ;
#14495=EDGE_LOOP ( 'NONE', ( #14813, #11537, #18045, #1283 ) ) ;
#14532=EDGE_LOOP ( 'NONE', ( #19013, #8952, #11029, #13776, #14979, #10488, #15923, #12584 ) ) ;
#14543=DIRECTION ( 'NONE',  ( -1.000000000000000000, -1.224646799147353207E-16, 0.000000000000000000 ) ) ;
#14589=ORIENTED_EDGE ( 'NONE', *, *, #170, .T. ) ;
#14609=DIRECTION ( 'NONE',  ( -1.000000000000000000, 1.224646799147353207E-16, 0.000000000000000000 ) ) ;
#14617=ORIENTED_EDGE ( 'NONE', *, *, #190, .F. ) ;
#14622=ORIENTED_EDGE ( 'NONE', *, *, #8356, .F. ) ;
#14639=DIRECTION ( 'NONE',  ( -1.000000000000000000, 1.224646799147353207E-16, 0.000000000000000000 ) ) ;
#14642=EDGE_CURVE ( 'NONE', #9172, #14916, #5866, .T. ) ;
#14653=CIRCLE ( 'NONE', #2491, 4.400000000000000355 ) ;
#14701=CARTESIAN_POINT ( 'NONE',  ( -36.00000000000000000, -4.400000000000000355, 5.388445916248354013E-16 ) ) ;
#14713=DIRECTION ( 'NONE',  ( 0.000000000000000000, 1.000000000000000000, 0.000000000000000000 ) ) ;
#14721=DIRECTION ( 'NONE',  ( 0.000000000000000000, -1.000000000000000000, 0.000000000000000000 ) ) ;
#14813=ORIENTED_EDGE ( 'NONE', *, *, #14642, .F. ) ;
#14909=ORIENTED_EDGE ( 'NONE', *, *, #170, .F. ) ;
#14911=DIRECTION ( 'NONE',  ( 0.000000000000000000, 0.000000000000000000, 1.000000000000000000 ) ) ;
#14916=VERTEX_POINT ( 'NONE', #11855 ) ;
#14929=AXIS2_PLACEMENT_3D ( 'NONE', #5540, #10067, #19153 ) ;
#14936=EDGE_LOOP ( 'NONE', ( #15121, #15173, #16369, #9675 ) ) ;
#14942=DIRECTION ( 'NONE',  ( -1.000000000000000000, -1.224646799147353207E-16, 0.000000000000000000 ) ) ;
#14945=VECTOR ( 'NONE', #3619, 1000.000000000000000 ) ;
#14976=ORIENTED_EDGE ( 'NONE', *, *, #19711, .T. ) ;
#14977=DIRECTION ( 'NONE',  ( -6.419766481290786633E-33, 1.000000000000000000, 0.000000000000000000 ) ) ;
#14979=ORIENTED_EDGE ( 'NONE', *, *, #19767, .T. ) ;
#15017=ADVANCED_FACE ( 'NONE', ( #14150 ), #9461, .T. ) ;
#15022=ORIENTED_EDGE ( 'NONE', *, *, #7346, .T. ) ;
#15029=CARTESIAN_POINT ( 'NONE',  ( -19.00000000000000355, 4.215373648918917304, 3.375000000000000888 ) ) ;
#15044=CARTESIAN_POINT ( 'NONE',  ( -41.99999999999999289, -2.000000000000001776, 5.000000000000000000 ) ) ;
#15058=DIRECTION ( 'NONE',  ( -1.000000000000000000, -6.419766481290786633E-33, 0.000000000000000000 ) ) ;
#15078=EDGE_LOOP ( 'NONE', ( #7210, #19446, #13707, #2232 ) ) ;
#15121=ORIENTED_EDGE ( 'NONE', *, *, #17923, .F. ) ;
#15128=DIRECTION ( 'NONE',  ( 0.000000000000000000, -1.000000000000000000, 0.000000000000000000 ) ) ;
#15134=ORIENTED_EDGE ( 'NONE', *, *, #19296, .T. ) ;
#15150=EDGE_CURVE ( 'NONE', #4430, #11599, #15803, .T. ) ;
#15173=ORIENTED_EDGE ( 'NONE', *, *, #18823, .T. ) ;
#15232=LINE ( 'NONE', #13, #17043 ) ;
#15255=AXIS2_PLACEMENT_3D ( 'NONE', #16793, #7958, #10779 ) ;
#15283=DIRECTION ( 'NONE',  ( 1.000000000000000000, 1.224646799147353207E-16, 0.000000000000000000 ) ) ;
#15333=CARTESIAN_POINT ( 'NONE',  ( -15.00000000000000355, -4.215373648918918192, 3.375000000000000888 ) ) ;
#15344=AXIS2_PLACEMENT_3D ( 'NONE', #19310, #13123, #5601 ) ;
#15379=DIRECTION ( 'NONE',  ( -1.000000000000000000, 1.224646799147353207E-16, 0.000000000000000000 ) ) ;
#15392=CIRCLE ( 'NONE', #11873, 8.000000000000000000 ) ;
#15409=AXIS2_PLACEMENT_3D ( 'NONE', #207, #8099, #5393 ) ;
#15430=EDGE_CURVE ( 'NONE', #3802, #12789, #6601, .T. ) ;
#15454=DIRECTION ( 'NONE',  ( 0.000000000000000000, -1.000000000000000000, 0.000000000000000000 ) ) ;
#15481=ORIENTED_EDGE ( 'NONE', *, *, #10428, .T. ) ;
#15483=FILL_AREA_STYLE_COLOUR ( '', #9078 ) ;
#15488=CARTESIAN_POINT ( 'NONE',  ( -41.99999999999999289, 4.999999999999998224, 2.000000000000000000 ) ) ;
#15493=CARTESIAN_POINT ( 'NONE',  ( -36.00000000000000000, -2.311115933264683024E-31, 0.000000000000000000 ) ) ;
#15503=DIRECTION ( 'NONE',  ( -1.000000000000000000, -1.224646799147353207E-16, -0.000000000000000000 ) ) ;
#15510=DIRECTION ( 'NONE',  ( 1.000000000000000000, 6.419766481290786633E-33, -0.000000000000000000 ) ) ;
#15512=DIRECTION ( 'NONE',  ( 0.000000000000000000, -1.000000000000000000, 0.000000000000000000 ) ) ;
#15533=DIRECTION ( 'NONE',  ( -9.559896011775280412E-17, -0.7806247497997995666, -0.6250000000000002220 ) ) ;
#15544=VERTEX_POINT ( 'NONE', #10930 ) ;
#15564=VECTOR ( 'NONE', #19637, 1000.000000000000000 ) ;
#15568=ADVANCED_FACE ( 'NONE', ( #8118 ), #14227, .T. ) ;
#15578=LINE ( 'NONE', #12475, #1508 ) ;
#15588=AXIS2_PLACEMENT_3D ( 'NONE', #12412, #4799, #10905 ) ;
#15589=DIRECTION ( 'NONE',  ( 0.000000000000000000, -1.000000000000000000, 0.000000000000000000 ) ) ;
#15631=CARTESIAN_POINT ( 'NONE',  ( -19.00000000000000355, -3.278623949159157558, -2.625000000000002220 ) ) ;
#15646=CARTESIAN_POINT ( 'NONE',  ( -41.99999999999999289, 1.999999999999998224, -5.000000000000000000 ) ) ;
#15652=DIRECTION ( 'NONE',  ( 0.000000000000000000, -3.552713678800500929E-15, 1.000000000000000000 ) ) ;
#15654=ORIENTED_EDGE ( 'NONE', *, *, #13594, .T. ) ;
#15677=FILL_AREA_STYLE ('',( #15483 ) ) ;
#15679=ORIENTED_EDGE ( 'NONE', *, *, #17156, .F. ) ;
#15693=LINE ( 'NONE', #14293, #18929 ) ;
#15696=ORIENTED_EDGE ( 'NONE', *, *, #9198, .T. ) ;
#15709=LINE ( 'NONE', #13810, #19710 ) ;
#15766=DIRECTION ( 'NONE',  ( -1.000000000000000000, -1.224646799147353207E-16, 0.000000000000000000 ) ) ;
#15784=DIRECTION ( 'NONE',  ( 9.559896011775280412E-17, 0.7806247497997995666, -0.6250000000000001110 ) ) ;
#15793=CARTESIAN_POINT ( 'NONE',  ( -11.00000000000000355, 4.898587196589412829E-16, 0.000000000000000000 ) ) ;
#15795=LINE ( 'NONE', #12694, #4860 ) ;
#15803=CIRCLE ( 'NONE', #11004, 4.400000000000000355 ) ;
#15816=ADVANCED_FACE ( 'NONE', ( #11912 ), #3204, .T. ) ;
#15870=DIRECTION ( 'NONE',  ( -0.000000000000000000, 0.000000000000000000, -1.000000000000000000 ) ) ;
#15923=ORIENTED_EDGE ( 'NONE', *, *, #11893, .F. ) ;
#15948=DIRECTION ( 'NONE',  ( 0.000000000000000000, -1.000000000000000000, 0.000000000000000000 ) ) ;
#15956=ORIENTED_EDGE ( 'NONE', *, *, #5764, .T. ) ;
#15992=CARTESIAN_POINT ( 'NONE',  ( -36.00000000000000000, 1.999999999999999112, 2.000000000000000000 ) ) ;
#16055=AXIS2_PLACEMENT_3D ( 'NONE', #10283, #2460, #8668 ) ;
#16140=DIRECTION ( 'NONE',  ( 1.000000000000000000, 6.419766481290786633E-33, -0.000000000000000000 ) ) ;
#16144=DIRECTION ( 'NONE',  ( -1.224646799147353207E-16, 1.000000000000000000, 0.000000000000000000 ) ) ;
#16145=LINE ( 'NONE', #11821, #13937 ) ;
#16210=CARTESIAN_POINT ( 'NONE',  ( -10.99900000000000233, -4.200000000000000178, 0.000000000000000000 ) ) ;
#16240=CYLINDRICAL_SURFACE ( 'NONE', #4919, 4.400000000000000355 ) ;
#16246=AXIS2_PLACEMENT_3D ( 'NONE', #9188, #4679, #13783 ) ;
#16254=LINE ( 'NONE', #17952, #3438 ) ;
#16285=CARTESIAN_POINT ( 'NONE',  ( -15.00000000000000355, 1.224646799147353454E-16, 0.000000000000000000 ) ) ;
#16291=CARTESIAN_POINT ( 'NONE',  ( -11.00000000000000355, 3.278623949159159778, 2.625000000000000888 ) ) ;
#16293=VERTEX_POINT ( 'NONE', #7621 ) ;
#16308=CYLINDRICAL_SURFACE ( 'NONE', #4497, 6.000000000000000888 ) ;
#16314=CARTESIAN_POINT ( 'NONE',  ( -19.00000000000000355, 4.898587196589412829E-16, 0.000000000000000000 ) ) ;
#16317=ORIENTED_EDGE ( 'NONE', *, *, #1887, .F. ) ;
#16347=CIRCLE ( 'NONE', #7706, 4.200000000000000178 ) ;
#16369=ORIENTED_EDGE ( 'NONE', *, *, #9391, .T. ) ;
#16375=CIRCLE ( 'NONE', #8392, 30.00000000000000000 ) ;
#16382=AXIS2_PLACEMENT_3D ( 'NONE', #6831, #17555, #13051 ) ;
#16391=ORIENTED_EDGE ( 'NONE', *, *, #13359, .F. ) ;
#16414=CARTESIAN_POINT ( 'NONE',  ( -19.00000000000000355, -3.434748899119118182, 2.750000000000001776 ) ) ;
#16421=CARTESIAN_POINT ( 'NONE',  ( -11.00000000000000355, -4.898587196589412829E-16, 0.000000000000000000 ) ) ;
#16444=ORIENTED_EDGE ( 'NONE', *, *, #7346, .F. ) ;
#16450=CARTESIAN_POINT ( 'NONE',  ( -19.00000000000000355, 4.898587196589412829E-16, 0.000000000000000000 ) ) ;
#16478=CIRCLE ( 'NONE', #10409, 4.200000000000000178 ) ;
#16512=ORIENTED_EDGE ( 'NONE', *, *, #8732, .F. ) ;
#16514=LINE ( 'NONE', #16715, #4296 ) ;
#16516=VERTEX_POINT ( 'NONE', #18532 ) ;
#16522=AXIS2_PLACEMENT_3D ( 'NONE', #3916, #16140, #17628 ) ;
#16560=CARTESIAN_POINT ( 'NONE',  ( -11.00000000000000355, -4.200000000000001066, 0.000000000000000000 ) ) ;
#16565=AXIS2_PLACEMENT_3D ( 'NONE', #15493, #483, #15589 ) ;
#16612=ORIENTED_EDGE ( 'NONE', *, *, #2002, .T. ) ;
#16626=DIRECTION ( 'NONE',  ( 5.011428603230760289E-33, -0.7806247497997995666, 0.6250000000000002220 ) ) ;
#16638=ADVANCED_FACE ( 'NONE', ( #920 ), #13224, .T. ) ;
#16642=CARTESIAN_POINT ( 'NONE',  ( -19.00000000000000355, -3.278623949159158890, 2.625000000000000888 ) ) ;
#16664=AXIS2_PLACEMENT_3D ( 'NONE', #10044, #16144, #14543 ) ;
#16668=AXIS2_PLACEMENT_3D ( 'NONE', #16450, #1534, #4631 ) ;
#16715=CARTESIAN_POINT ( 'NONE',  ( -11.00000000000000355, -3.278623949159158446, -2.625000000000002220 ) ) ;
#16724=AXIS2_PLACEMENT_3D ( 'NONE', #17428, #9833, #6230 ) ;
#16739=EDGE_CURVE ( 'NONE', #17554, #2370, #7997, .T. ) ;
#16751=ORIENTED_EDGE ( 'NONE', *, *, #527, .F. ) ;
#16787=CARTESIAN_POINT ( 'NONE',  ( -41.99999999999999289, -5.000000000000001776, 5.000000000000000000 ) ) ;
#16793=CARTESIAN_POINT ( 'NONE',  ( -11.00000000000000355, 4.898587196589412829E-16, 0.000000000000000000 ) ) ;
#16831=EDGE_LOOP ( 'NONE', ( #3312, #15022, #12985, #2247 ) ) ;
#16858=CARTESIAN_POINT ( 'NONE',  ( -11.00000000000000355, -4.215373648918917304, -3.375000000000002665 ) ) ;
#16867=SHAPE_DEFINITION_REPRESENTATION ( #767, #12077 ) ;
#16897=EDGE_CURVE ( 'NONE', #11950, #12571, #5189, .T. ) ;
#16904=ORIENTED_EDGE ( 'NONE', *, *, #19561, .T. ) ;
#16926=VERTEX_POINT ( 'NONE', #5969 ) ;
#16974=EDGE_CURVE ( 'NONE', #3279, #12070, #973, .T. ) ;
#16982=VERTEX_POINT ( 'NONE', #8989 ) ;
#16993=CIRCLE ( 'NONE', #7377, 4.400000000000000355 ) ;
#17011=VECTOR ( 'NONE', #13889, 1000.000000000000114 ) ;
#17015=DIRECTION ( 'NONE',  ( 1.000000000000000000, 6.419766481290786633E-33, -0.000000000000000000 ) ) ;
#17017=CYLINDRICAL_SURFACE ( 'NONE', #15409, 3.000000000000000000 ) ;
#17019=EDGE_LOOP ( 'NONE', ( #19343, #3769, #843, #1870, #9840, #3442, #19491, #644 ) ) ;
#17035=ORIENTED_EDGE ( 'NONE', *, *, #5034, .F. ) ;
#17039=VERTEX_POINT ( 'NONE', #5676 ) ;
#17043=VECTOR ( 'NONE', #16626, 1000.000000000000000 ) ;
#17048=FACE_OUTER_BOUND ( 'NONE', #14368, .T. ) ;
#17083=ORIENTED_EDGE ( 'NONE', *, *, #19029, .T. ) ;
#17118=ORIENTED_EDGE ( 'NONE', *, *, #5034, .T. ) ;
#17129=CYLINDRICAL_SURFACE ( 'NONE', #11011, 4.400000000000000355 ) ;
#17150=CARTESIAN_POINT ( 'NONE',  ( -36.00000000000000000, 1.224646799147351975E-16, 0.000000000000000000 ) ) ;
#17151=DIRECTION ( 'NONE',  ( 1.000000000000000000, 1.224646799147353207E-16, -0.000000000000000000 ) ) ;
#17156=EDGE_CURVE ( 'NONE', #16926, #4917, #13888, .T. ) ;
#17170=AXIS2_PLACEMENT_3D ( 'NONE', #12586, #7867, #4777 ) ;
#17176=EDGE_CURVE ( 'NONE', #9264, #6659, #10240, .T. ) ;
#17203=DIRECTION ( 'NONE',  ( -6.419766481290786633E-33, 1.000000000000000000, 0.000000000000000000 ) ) ;
#17213=LINE ( 'NONE', #13916, #19738 ) ;
#17230=AXIS2_PLACEMENT_3D ( 'NONE', #6542, #17373, #12673 ) ;
#17244=CARTESIAN_POINT ( 'NONE',  ( -11.00000000000000355, -4.898587196589412829E-16, 0.000000000000000000 ) ) ;
#17288=VERTEX_POINT ( 'NONE', #2739 ) ;
#17296=DIRECTION ( 'NONE',  ( -1.000000000000000000, -6.419766481290786633E-33, 0.000000000000000000 ) ) ;
#17297=DIRECTION ( 'NONE',  ( 0.000000000000000000, -1.000000000000000000, 0.000000000000000000 ) ) ;
#17331=ADVANCED_FACE ( 'NONE', ( #9828 ), #16308, .T. ) ;
#17349=AXIS2_PLACEMENT_3D ( 'NONE', #16787, #9178, #15283 ) ;
#17350=DIRECTION ( 'NONE',  ( 1.000000000000000000, 6.419766481290786633E-33, -0.000000000000000000 ) ) ;
#17373=DIRECTION ( 'NONE',  ( 0.000000000000000000, 0.000000000000000000, 1.000000000000000000 ) ) ;
#17417=AXIS2_PLACEMENT_3D ( 'NONE', #7887, #1892, #17297 ) ;
#17428=CARTESIAN_POINT ( 'NONE',  ( 0.000000000000000000, 0.000000000000000000, 0.000000000000000000 ) ) ;
#17448=CYLINDRICAL_SURFACE ( 'NONE', #3294, 4.200000000000000178 ) ;
#17453=DIRECTION ( 'NONE',  ( 1.000000000000000000, 1.224646799147353207E-16, -0.000000000000000000 ) ) ;
#17491=FACE_OUTER_BOUND ( 'NONE', #15078, .T. ) ;
#17536=CARTESIAN_POINT ( 'NONE',  ( -22.50000000000000711, 21.04737509655562988, -2.577560054245056178E-15 ) ) ;
#17547=AXIS2_PLACEMENT_3D ( 'NONE', #12664, #15766, #2347 ) ;
#17549=DIRECTION ( 'NONE',  ( 0.000000000000000000, 1.000000000000000000, 0.000000000000000000 ) ) ;
#17554=VERTEX_POINT ( 'NONE', #14087 ) ;
#17555=DIRECTION ( 'NONE',  ( -1.000000000000000000, -6.419766481290786633E-33, 0.000000000000000000 ) ) ;
#17628=DIRECTION ( 'NONE',  ( 0.000000000000000000, 1.000000000000000000, 0.000000000000000000 ) ) ;
#17637=AXIS2_PLACEMENT_3D ( 'NONE', #3105, #18510, #4907 ) ;
#17642=ORIENTED_EDGE ( 'NONE', *, *, #5496, .T. ) ;
#17658=FACE_OUTER_BOUND ( 'NONE', #11344, .T. ) ;
#17678=AXIS2_PLACEMENT_3D ( 'NONE', #8163, #573, #6644 ) ;
#17691=CARTESIAN_POINT ( 'NONE',  ( -30.00000000000000000, 4.400000000000000355, 0.000000000000000000 ) ) ;
#17723=AXIS2_PLACEMENT_3D ( 'NONE', #16314, #913, #14911 ) ;
#17728=ADVANCED_FACE ( 'NONE', ( #17491 ), #3780, .F. ) ;
#17767=ADVANCED_FACE ( 'NONE', ( #9901 ), #10363, .F. ) ;
#17769=ORIENTED_EDGE ( 'NONE', *, *, #11530, .F. ) ;
#17771=CARTESIAN_POINT ( 'NONE',  ( -11.00000000000000355, -4.898587196589412829E-16, 0.000000000000000000 ) ) ;
#17802=EDGE_LOOP ( 'NONE', ( #10216, #7307, #13333, #12042 ) ) ;
#17815=EDGE_CURVE ( 'NONE', #10991, #9264, #1246, .T. ) ;
#17825=CARTESIAN_POINT ( 'NONE',  ( -19.00000000000000355, -4.898587196589412829E-16, 0.000000000000000000 ) ) ;
#17843=EDGE_LOOP ( 'NONE', ( #12838, #7753 ) ) ;
#17849=CARTESIAN_POINT ( 'NONE',  ( -36.00000000000000000, -2.311115933264683024E-31, 0.000000000000000000 ) ) ;
#17885=ADVANCED_FACE ( 'NONE', ( #12154 ), #4641, .T. ) ;
#17923=EDGE_CURVE ( 'NONE', #6659, #5646, #18543, .T. ) ;
#17936=VERTEX_POINT ( 'NONE', #16858 ) ;
#17943=VERTEX_POINT ( 'NONE', #10848 ) ;
#17952=CARTESIAN_POINT ( 'NONE',  ( -11.00000000000000355, 4.215373648918918192, 3.375000000000000888 ) ) ;
#17960=DIRECTION ( 'NONE',  ( -7.654042494670959086E-17, 0.6250000000000002220, -0.7806247497997996776 ) ) ;
#17961=CIRCLE ( 'NONE', #10937, 4.400000000000001243 ) ;
#17967=VERTEX_POINT ( 'NONE', #7734 ) ;
#18018=ORIENTED_EDGE ( 'NONE', *, *, #385, .T. ) ;
#18045=ORIENTED_EDGE ( 'NONE', *, *, #12251, .T. ) ;
#18075=AXIS2_PLACEMENT_3D ( 'NONE', #6510, #4633, #12638 ) ;
#18080=CARTESIAN_POINT ( 'NONE',  ( -11.00000000000000355, 4.215373648918918192, 3.375000000000000888 ) ) ;
#18095=CARTESIAN_POINT ( 'NONE',  ( -41.99999999999999289, -2.000000000000001776, -2.000000000000000000 ) ) ;
#18107=EDGE_CURVE ( 'NONE', #14054, #6506, #13772, .T. ) ;
#18145=FACE_OUTER_BOUND ( 'NONE', #14007, .T. ) ;
#18156=EDGE_CURVE ( 'NONE', #4917, #5485, #16993, .T. ) ;
#18199=CARTESIAN_POINT ( 'NONE',  ( -15.00000000000000355, 3.434748899119118626, 2.750000000000001332 ) ) ;
#18224=CYLINDRICAL_SURFACE ( 'NONE', #17637, 3.000000000000000000 ) ;
#18281=PLANE ( 'NONE',  #17349 ) ;
#18282=ADVANCED_FACE ( 'NONE', ( #2516 ), #8624, .T. ) ;
#18337=ORIENTED_EDGE ( 'NONE', *, *, #16739, .F. ) ;
#18340=CIRCLE ( 'NONE', #467, 5.400000000000000355 ) ;
#18351=CARTESIAN_POINT ( 'NONE',  ( -36.00000000000000000, 4.999999999999999112, 5.000000000000000000 ) ) ;
#18392=VERTEX_POINT ( 'NONE', #18619 ) ;
#18434=EDGE_CURVE ( 'NONE', #3616, #2009, #16347, .T. ) ;
#18436=DIRECTION ( 'NONE',  ( -1.000000000000000000, -6.419766481290786633E-33, 0.000000000000000000 ) ) ;
#18450=CARTESIAN_POINT ( 'NONE',  ( -19.00000000000000355, 4.898587196589412829E-16, 0.000000000000000000 ) ) ;
#18454=ORIENTED_EDGE ( 'NONE', *, *, #11619, .F. ) ;
#18480=CARTESIAN_POINT ( 'NONE',  ( -11.00000000000000355, -4.898587196589412829E-16, 0.000000000000000000 ) ) ;
#18502=EDGE_CURVE ( 'NONE', #6506, #14054, #15392, .T. ) ;
#18510=DIRECTION ( 'NONE',  ( 1.000000000000000000, 1.224646799147353207E-16, 0.000000000000000000 ) ) ;
#18531=EDGE_LOOP ( 'NONE', ( #17035, #11602, #315, #18817 ) ) ;
#18532=CARTESIAN_POINT ( 'NONE',  ( -15.00000000000000355, 4.215373648918916416, -3.375000000000002665 ) ) ;
#18540=AXIS2_PLACEMENT_3D ( 'NONE', #1581, #7669, #13753 ) ;
#18543=LINE ( 'NONE', #18351, #4508 ) ;
#18601=EDGE_LOOP ( 'NONE', ( #14350, #516, #19368, #11739 ) ) ;
#18616=EDGE_CURVE ( 'NONE', #4963, #18392, #11264, .T. ) ;
#18617=CLOSED_SHELL ( 'NONE', ( #2130, #1693, #4323, #18282, #12911, #15816, #9922, #3638, #10926, #2933, #8946, #640, #17728, #12028, #6700, #17767, #10455, #6658, #4277, #15568, #17885, #9702, #13108, #8066, #17331, #14317, #5176, #7260, #413, #15017, #7153, #8168, #13924, #19275, #16638, #19650, #14, #371 ) ) ;
#18619=CARTESIAN_POINT ( 'NONE',  ( -15.00000000000000355, -3.434748899119118626, 2.750000000000001332 ) ) ;
#18633=CIRCLE ( 'NONE', #10024, 4.200000000000000178 ) ;
#18643=CYLINDRICAL_SURFACE ( 'NONE', #3940, 3.000000000000000000 ) ;
#18656=DIRECTION ( 'NONE',  ( 0.000000000000000000, -1.000000000000000000, 0.000000000000000000 ) ) ;
#18672=PRESENTATION_STYLE_ASSIGNMENT (( #3469 ) ) ;
#18699=CARTESIAN_POINT ( 'NONE',  ( -19.00000000000000355, -3.278623949159157558, -2.625000000000002220 ) ) ;
#18713=CARTESIAN_POINT ( 'NONE',  ( -15.00000000000000355, 1.224646799147353454E-16, 0.000000000000000000 ) ) ;
#18733=LINE ( 'NONE', #5121, #1469 ) ;
#18741=DIRECTION ( 'NONE',  ( -1.000000000000000000, 1.224646799147353207E-16, 0.000000000000000000 ) ) ;
#18745=LINE ( 'NONE', #5039, #4334 ) ;
#18763=AXIS2_PLACEMENT_3D ( 'NONE', #5216, #11335, #14721 ) ;
#18817=ORIENTED_EDGE ( 'NONE', *, *, #12251, .F. ) ;
#18823=EDGE_CURVE ( 'NONE', #6659, #17967, #15795, .T. ) ;
#18839=ORIENTED_EDGE ( 'NONE', *, *, #11619, .T. ) ;
#18877=ORIENTED_EDGE ( 'NONE', *, *, #13795, .T. ) ;
#18882=EDGE_LOOP ( 'NONE', ( #14622, #10638 ) ) ;
#18900=CIRCLE ( 'NONE', #2278, 4.200000000000000178 ) ;
#18908=ORIENTED_EDGE ( 'NONE', *, *, #12486, .T. ) ;
#18910=DIRECTION ( 'NONE',  ( 0.000000000000000000, 1.000000000000000000, 0.000000000000000000 ) ) ;
#18918=CARTESIAN_POINT ( 'NONE',  ( -15.00000000000000355, 1.224646799147353454E-16, 0.000000000000000000 ) ) ;
#18929=VECTOR ( 'NONE', #12403, 1000.000000000000114 ) ;
#18930=STYLED_ITEM ( 'NONE', ( #11262 ), #9200 ) ;
#18937=EDGE_CURVE ( 'NONE', #4963, #4614, #15693, .T. ) ;
#18938=PLANE ( 'NONE',  #5828 ) ;
#18974=EDGE_LOOP ( 'NONE', ( #1867, #3759, #19528, #16512 ) ) ;
#19004=EDGE_CURVE ( 'NONE', #12710, #4605, #11488, .T. ) ;
#19008=ORIENTED_EDGE ( 'NONE', *, *, #504, .F. ) ;
#19013=ORIENTED_EDGE ( 'NONE', *, *, #4824, .F. ) ;
#19014=DIRECTION ( 'NONE',  ( 1.000000000000000000, 6.419766481290786633E-33, -0.000000000000000000 ) ) ;
#19024=ORIENTED_EDGE ( 'NONE', *, *, #16974, .F. ) ;
#19029=EDGE_CURVE ( 'NONE', #16926, #3728, #17961, .T. ) ;
#19046=DIRECTION ( 'NONE',  ( 0.000000000000000000, 1.776356839400250465E-15, 1.000000000000000000 ) ) ;
#19153=DIRECTION ( 'NONE',  ( 0.000000000000000000, -1.000000000000000000, 0.000000000000000000 ) ) ;
#19166=ORIENTED_EDGE ( 'NONE', *, *, #4561, .F. ) ;
#19225=VECTOR ( 'NONE', #1395, 1000.000000000000000 ) ;
#19246=CARTESIAN_POINT ( 'NONE',  ( -11.00000000000000355, -3.278623949159159778, 2.625000000000000888 ) ) ;
#19253=CIRCLE ( 'NONE', #2010, 3.000000000000000000 ) ;
#19266=EDGE_CURVE ( 'NONE', #5485, #4917, #12555, .T. ) ;
#19270=DIRECTION ( 'NONE',  ( 1.000000000000000000, 6.419766481290786633E-33, -0.000000000000000000 ) ) ;
#19275=ADVANCED_FACE ( 'NONE', ( #12176 ), #18281, .T. ) ;
#19277=DIRECTION ( 'NONE',  ( -9.559896011775280412E-17, 0.7806247497997995666, -0.6250000000000002220 ) ) ;
#19296=EDGE_CURVE ( 'NONE', #3019, #16293, #6347, .T. ) ;
#19297=CIRCLE ( 'NONE', #10055, 3.000000000000000000 ) ;
#19310=CARTESIAN_POINT ( 'NONE',  ( -41.99999999999999289, -5.000000000000001776, -5.000000000000000000 ) ) ;
#19315=DIRECTION ( 'NONE',  ( 0.000000000000000000, 1.776356839400250465E-15, 1.000000000000000000 ) ) ;
#19335=EDGE_LOOP ( 'NONE', ( #1882, #9233, #18877, #18908, #7447, #11569, #96, #7041 ) ) ;
#19338=CARTESIAN_POINT ( 'NONE',  ( -15.00000000000000355, -8.000000000000000000, 9.797174393178825657E-16 ) ) ;
#19343=ORIENTED_EDGE ( 'NONE', *, *, #11980, .F. ) ;
#19368=ORIENTED_EDGE ( 'NONE', *, *, #11980, .T. ) ;
#19375=VECTOR ( 'NONE', #7369, 1000.000000000000000 ) ;
#19382=ORIENTED_EDGE ( 'NONE', *, *, #18937, .T. ) ;
#19398=EDGE_CURVE ( 'NONE', #17936, #14330, #11172, .T. ) ;
#19433=CIRCLE ( 'NONE', #12737, 6.000000000000000888 ) ;
#19434=DIRECTION ( 'NONE',  ( 0.000000000000000000, -1.000000000000000000, 0.000000000000000000 ) ) ;
#19446=ORIENTED_EDGE ( 'NONE', *, *, #12930, .F. ) ;
#19460=DIRECTION ( 'NONE',  ( -1.000000000000000000, 1.224646799147353207E-16, 0.000000000000000000 ) ) ;
#19466=ORIENTED_EDGE ( 'NONE', *, *, #7560, .F. ) ;
#19489=CARTESIAN_POINT ( 'NONE',  ( -41.99999999999999289, 1.999999999999998224, -2.000000000000000000 ) ) ;
#19491=ORIENTED_EDGE ( 'NONE', *, *, #9391, .F. ) ;
#19511=CARTESIAN_POINT ( 'NONE',  ( -19.00000000000000355, 3.434748899119117294, -2.750000000000002220 ) ) ;
#19528=ORIENTED_EDGE ( 'NONE', *, *, #7757, .F. ) ;
#19538=EDGE_CURVE ( 'NONE', #3728, #5485, #10076, .T. ) ;
#19561=EDGE_CURVE ( 'NONE', #530, #3222, #410, .T. ) ;
#19563=DIRECTION ( 'NONE',  ( 0.000000000000000000, -1.000000000000000000, 0.000000000000000000 ) ) ;
#19587=UNCERTAINTY_MEASURE_WITH_UNIT (LENGTH_MEASURE( 1.000000000000000082E-05 ), #4281, 'distance_accuracy_value', 'NONE');
#19606=DIRECTION ( 'NONE',  ( 1.000000000000000000, 6.419766481290786633E-33, -0.000000000000000000 ) ) ;
#19637=DIRECTION ( 'NONE',  ( 1.000000000000000000, 6.419766481290786633E-33, -0.000000000000000000 ) ) ;
#19650=ADVANCED_FACE ( 'NONE', ( #5843, #4354 ), #4451, .F. ) ;
#19702=ORIENTED_EDGE ( 'NONE', *, *, #19004, .T. ) ;
#19710=VECTOR ( 'NONE', #17015, 1000.000000000000000 ) ;
#19711=EDGE_CURVE ( 'NONE', #3728, #16926, #6162, .T. ) ;
#19728=EDGE_LOOP ( 'NONE', ( #16751, #4556, #610, #708, #19702, #13158 ) ) ;
#19734=DIRECTION ( 'NONE',  ( 0.000000000000000000, -1.000000000000000000, 0.000000000000000000 ) ) ;
#19738=VECTOR ( 'NONE', #4808, 1000.000000000000000 ) ;
#19750=CARTESIAN_POINT ( 'NONE',  ( -30.00000000000000000, -1.925929944387235853E-31, 0.000000000000000000 ) ) ;
#19765=ORIENTED_EDGE ( 'NONE', *, *, #12844, .T. ) ;
#19767=EDGE_CURVE ( 'NONE', #17943, #4963, #2015, .T. ) ;
#19768=DIRECTION ( 'NONE',  ( -1.000000000000000000, -6.419766481290786633E-33, 0.000000000000000000 ) ) ;
#19773=CARTESIAN_POINT ( 'NONE',  ( -15.00000000000000355, -3.434748899119117294, -2.750000000000002220 ) ) ;
#19775=EDGE_LOOP ( 'NONE', ( #6175, #14589, #4463, #13419 ) ) ;
ENDSEC;
END-ISO-10303-21;
